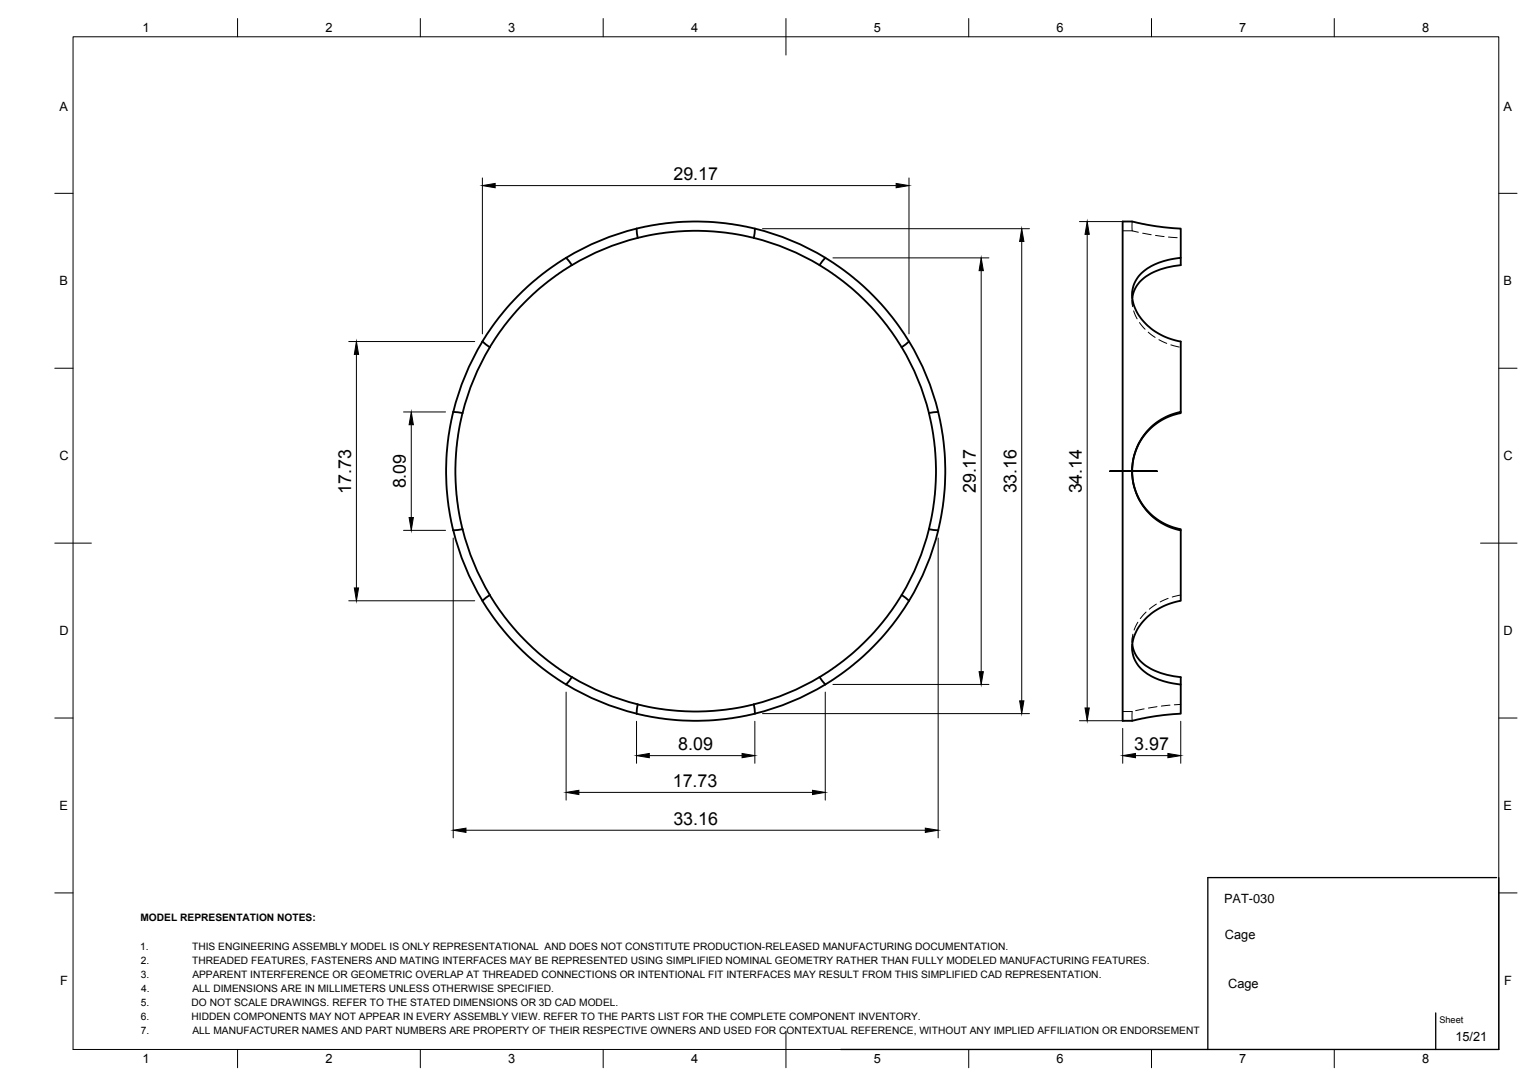
ISO-10303-21;
HEADER;
/* Generated by software containing ST-Developer
 * from STEP Tools, Inc. (www.steptools.com) 
 */

FILE_DESCRIPTION(
/* description */ ('Double-bearing flanged cartridge'),
/* implementation_level */ '2;1');

FILE_NAME(
/* name */ 'Cage.step',
/* time_stamp */ '2026-10-28T03:26:40-07:00',
/* author */ (''),
/* organization */ (''),
/* preprocessor_version */ 'ST-DEVELOPER v20.2',
/* originating_system */ 'Autodesk Translation Framework v15.17.0.0',
/* authorisation */ '');

FILE_SCHEMA (('AUTOMOTIVE_DESIGN { 1 0 10303 214 3 1 1 }'));
ENDSEC;

DATA;
#10=MECHANICAL_DESIGN_GEOMETRIC_PRESENTATION_REPRESENTATION('',(#201),#5535);
#116=B_SPLINE_CURVE_WITH_KNOTS('',3,(#3902,#3903,#3904,#3905,#3906,#3907,
#3908,#3909,#3910,#3911,#3912,#3913,#3914,#3915,#3916,#3917,#3918,#3919,
#3920,#3921,#3922,#3923),.UNSPECIFIED.,.F.,.F.,(4,2,2,2,2,2,2,2,2,2,4),
(0.0789094028588958,0.210573405340968,0.315860108011452,0.421146810681936,
0.522142632548711,0.623138454415485,0.72413427628226,0.825130098149035,
0.930416800819519,1.03570350349,1.16736750597208),.UNSPECIFIED.);
#117=B_SPLINE_CURVE_WITH_KNOTS('',3,(#3927,#3928,#3929,#3930,#3931,#3932,
#3933,#3934,#3935,#3936,#3937,#3938,#3939,#3940,#3941,#3942,#3943,#3944,
#3945,#3946,#3947,#3948),.UNSPECIFIED.,.F.,.F.,(4,2,2,2,2,2,2,2,2,2,4),
(0.0774793363974613,0.142088896491891,0.284177792983782,0.411119756996526,
0.514392970548519,0.617666184100513,0.720939397652506,0.8242126112045,0.951154575217244,
1.09324347170913,1.15785303180356),.UNSPECIFIED.);
#118=B_SPLINE_CURVE_WITH_KNOTS('',3,(#3954,#3955,#3956,#3957,#3958,#3959,
#3960,#3961,#3962,#3963,#3964,#3965,#3966,#3967,#3968,#3969,#3970,#3971,
#3972,#3973,#3974,#3975),.UNSPECIFIED.,.F.,.F.,(4,2,2,2,2,2,2,2,2,2,4),
(0.0774793363974613,0.142088896491891,0.284177792983782,0.411119756996525,
0.514392970548519,0.617666184100513,0.720939397652506,0.8242126112045,0.951154575217243,
1.09324347170913,1.15785303180356),.UNSPECIFIED.);
#119=B_SPLINE_CURVE_WITH_KNOTS('',3,(#3979,#3980,#3981,#3982,#3983,#3984,
#3985,#3986,#3987,#3988,#3989,#3990,#3991,#3992,#3993,#3994,#3995,#3996,
#3997,#3998,#3999,#4000),.UNSPECIFIED.,.F.,.F.,(4,2,2,2,2,2,2,2,2,2,4),
(0.0774793363974614,0.142088896491891,0.284177792983781,0.411119756996525,
0.514392970548519,0.617666184100512,0.720939397652506,0.824212611204499,
0.951154575217243,1.09324347170913,1.15785303180356),.UNSPECIFIED.);
#120=B_SPLINE_CURVE_WITH_KNOTS('',3,(#4004,#4005,#4006,#4007,#4008,#4009,
#4010,#4011,#4012,#4013,#4014,#4015),.UNSPECIFIED.,.F.,.F.,(4,2,2,2,2,4),
(0.0774793363974613,0.142088896491891,0.284177792983781,0.411119756996525,
0.514392970548519,0.617666184100512),.UNSPECIFIED.);
#121=B_SPLINE_CURVE_WITH_KNOTS('',3,(#4020,#4021,#4022,#4023,#4024,#4025,
#4026,#4027,#4028,#4029,#4030,#4031),.UNSPECIFIED.,.F.,.F.,(4,2,2,2,2,4),
(0.617666184100512,0.720939397652506,0.824212611204499,0.951154575217243,
1.09324347170913,1.15785303180356),.UNSPECIFIED.);
#122=B_SPLINE_CURVE_WITH_KNOTS('',3,(#4035,#4036,#4037,#4038,#4039,#4040,
#4041,#4042,#4043,#4044,#4045,#4046,#4047,#4048,#4049,#4050,#4051,#4052,
#4053,#4054,#4055,#4056),.UNSPECIFIED.,.F.,.F.,(4,2,2,2,2,2,2,2,2,2,4),
(0.0774793363974613,0.142088896491891,0.284177792983782,0.411119756996526,
0.514392970548519,0.617666184100513,0.720939397652507,0.8242126112045,0.951154575217245,
1.09324347170914,1.15785303180356),.UNSPECIFIED.);
#123=B_SPLINE_CURVE_WITH_KNOTS('',3,(#4060,#4061,#4062,#4063,#4064,#4065,
#4066,#4067,#4068,#4069,#4070,#4071,#4072,#4073,#4074,#4075,#4076,#4077,
#4078,#4079,#4080,#4081),.UNSPECIFIED.,.F.,.F.,(4,2,2,2,2,2,2,2,2,2,4),
(0.0774793363974613,0.142088896491891,0.284177792983782,0.411119756996526,
0.514392970548519,0.617666184100513,0.720939397652506,0.824212611204499,
0.951154575217243,1.09324347170913,1.15785303180356),.UNSPECIFIED.);
#124=B_SPLINE_CURVE_WITH_KNOTS('',3,(#4085,#4086,#4087,#4088,#4089,#4090,
#4091,#4092,#4093,#4094,#4095,#4096,#4097,#4098,#4099,#4100,#4101,#4102,
#4103,#4104,#4105,#4106),.UNSPECIFIED.,.F.,.F.,(4,2,2,2,2,2,2,2,2,2,4),
(0.0774793363974613,0.142088896491891,0.284177792983782,0.411119756996526,
0.514392970548519,0.617666184100513,0.720939397652506,0.8242126112045,0.951154575217244,
1.09324347170913,1.15785303180356),.UNSPECIFIED.);
#125=B_SPLINE_CURVE_WITH_KNOTS('',3,(#4110,#4111,#4112,#4113,#4114,#4115,
#4116,#4117,#4118,#4119,#4120,#4121,#4122,#4123,#4124,#4125,#4126,#4127,
#4128,#4129,#4130,#4131),.UNSPECIFIED.,.F.,.F.,(4,2,2,2,2,2,2,2,2,2,4),
(0.0774793363974613,0.142088896491891,0.284177792983782,0.411119756996526,
0.514392970548519,0.617666184100513,0.720939397652506,0.8242126112045,0.951154575217243,
1.09324347170913,1.15785303180356),.UNSPECIFIED.);
#126=B_SPLINE_CURVE_WITH_KNOTS('',3,(#4139,#4140,#4141,#4142,#4143,#4144,
#4145,#4146,#4147,#4148,#4149,#4150,#4151,#4152,#4153,#4154,#4155,#4156,
#4157,#4158,#4159,#4160),.UNSPECIFIED.,.F.,.F.,(4,2,2,2,2,2,2,2,2,2,4),
(0.0789094028588958,0.210573405340968,0.315860108011452,0.421146810681936,
0.522142632548711,0.623138454415485,0.72413427628226,0.825130098149035,
0.930416800819519,1.03570350349,1.16736750597208),.UNSPECIFIED.);
#127=B_SPLINE_CURVE_WITH_KNOTS('',3,(#4168,#4169,#4170,#4171,#4172,#4173,
#4174,#4175,#4176,#4177,#4178,#4179,#4180,#4181,#4182,#4183,#4184,#4185,
#4186,#4187,#4188,#4189),.UNSPECIFIED.,.F.,.F.,(4,2,2,2,2,2,2,2,2,2,4),
(0.0789094028588958,0.210573405340969,0.315860108011453,0.421146810681937,
0.522142632548712,0.623138454415486,0.724134276282261,0.825130098149035,
0.930416800819519,1.03570350349,1.16736750597208),.UNSPECIFIED.);
#128=B_SPLINE_CURVE_WITH_KNOTS('',3,(#4198,#4199,#4200,#4201,#4202,#4203,
#4204,#4205,#4206,#4207,#4208,#4209),.UNSPECIFIED.,.F.,.F.,(4,2,2,2,2,4),
(0.0789094028588958,0.210573405340968,0.315860108011452,0.421146810681937,
0.522142632548711,0.623138454415486),.UNSPECIFIED.);
#129=B_SPLINE_CURVE_WITH_KNOTS('',3,(#4211,#4212,#4213,#4214,#4215,#4216,
#4217,#4218,#4219,#4220,#4221,#4222),.UNSPECIFIED.,.F.,.F.,(4,2,2,2,2,4),
(0.623138454415486,0.72413427628226,0.825130098149035,0.930416800819519,
1.03570350349,1.16736750597208),.UNSPECIFIED.);
#130=B_SPLINE_CURVE_WITH_KNOTS('',3,(#4229,#4230,#4231,#4232,#4233,#4234,
#4235,#4236,#4237,#4238,#4239,#4240,#4241,#4242,#4243,#4244,#4245,#4246,
#4247,#4248,#4249,#4250),.UNSPECIFIED.,.F.,.F.,(4,2,2,2,2,2,2,2,2,2,4),
(0.0789094028588958,0.210573405340968,0.315860108011452,0.421146810681936,
0.522142632548711,0.623138454415486,0.72413427628226,0.825130098149035,
0.930416800819519,1.03570350349,1.16736750597208),.UNSPECIFIED.);
#131=B_SPLINE_CURVE_WITH_KNOTS('',3,(#4258,#4259,#4260,#4261,#4262,#4263,
#4264,#4265,#4266,#4267,#4268,#4269,#4270,#4271,#4272,#4273,#4274,#4275,
#4276,#4277,#4278,#4279),.UNSPECIFIED.,.F.,.F.,(4,2,2,2,2,2,2,2,2,2,4),
(0.0789094028588957,0.210573405340968,0.315860108011452,0.421146810681936,
0.522142632548711,0.623138454415485,0.72413427628226,0.825130098149035,
0.930416800819519,1.03570350349,1.16736750597207),.UNSPECIFIED.);
#132=B_SPLINE_CURVE_WITH_KNOTS('',3,(#4287,#4288,#4289,#4290,#4291,#4292,
#4293,#4294,#4295,#4296,#4297,#4298,#4299,#4300,#4301,#4302,#4303,#4304,
#4305,#4306,#4307,#4308),.UNSPECIFIED.,.F.,.F.,(4,2,2,2,2,2,2,2,2,2,4),
(0.0789094028588958,0.210573405340968,0.315860108011452,0.421146810681936,
0.522142632548711,0.623138454415486,0.72413427628226,0.825130098149035,
0.930416800819519,1.03570350349,1.16736750597208),.UNSPECIFIED.);
#133=B_SPLINE_CURVE_WITH_KNOTS('',3,(#4317,#4318,#4319,#4320,#4321,#4322,
#4323,#4324,#4325,#4326,#4327,#4328,#4329,#4330,#4331,#4332,#4333,#4334,
#4335,#4336,#4337,#4338),.UNSPECIFIED.,.F.,.F.,(4,2,2,2,2,2,2,2,2,2,4),
(0.0789094028588958,0.210573405340968,0.315860108011452,0.421146810681936,
0.522142632548711,0.623138454415485,0.72413427628226,0.825130098149035,
0.930416800819519,1.03570350349,1.16736750597208),.UNSPECIFIED.);
#144=SPHERICAL_SURFACE('',#2624,0.412776);
#145=SPHERICAL_SURFACE('',#2640,0.412776);
#146=SPHERICAL_SURFACE('',#2645,0.412776);
#147=SPHERICAL_SURFACE('',#2650,0.412776);
#148=SPHERICAL_SURFACE('',#2655,0.412776);
#149=SPHERICAL_SURFACE('',#2660,0.412776);
#150=SPHERICAL_SURFACE('',#2665,0.412776);
#151=SPHERICAL_SURFACE('',#2673,0.412776);
#166=SHAPE_REPRESENTATION_RELATIONSHIP('SRR','None',#5608,#180);
#180=ADVANCED_BREP_SHAPE_REPRESENTATION('',(#223),#5524);
#201=STYLED_ITEM('',(#5764),#223);
#223=MANIFOLD_SOLID_BREP('Continuous crown cage',#2335);
#257=FACE_BOUND('',#604,.T.);
#316=PLANE('',#2637);
#317=PLANE('',#2642);
#318=PLANE('',#2647);
#319=PLANE('',#2652);
#320=PLANE('',#2657);
#321=PLANE('',#2662);
#322=PLANE('',#2671);
#323=PLANE('',#2675);
#324=PLANE('',#2676);
#413=FACE_OUTER_BOUND('',#586,.T.);
#414=FACE_OUTER_BOUND('',#587,.T.);
#415=FACE_OUTER_BOUND('',#588,.T.);
#416=FACE_OUTER_BOUND('',#589,.T.);
#417=FACE_OUTER_BOUND('',#590,.T.);
#418=FACE_OUTER_BOUND('',#591,.T.);
#419=FACE_OUTER_BOUND('',#592,.T.);
#420=FACE_OUTER_BOUND('',#593,.T.);
#421=FACE_OUTER_BOUND('',#594,.T.);
#422=FACE_OUTER_BOUND('',#595,.T.);
#423=FACE_OUTER_BOUND('',#596,.T.);
#424=FACE_OUTER_BOUND('',#597,.T.);
#425=FACE_OUTER_BOUND('',#598,.T.);
#426=FACE_OUTER_BOUND('',#599,.T.);
#427=FACE_OUTER_BOUND('',#600,.T.);
#428=FACE_OUTER_BOUND('',#601,.T.);
#429=FACE_OUTER_BOUND('',#602,.T.);
#430=FACE_OUTER_BOUND('',#603,.T.);
#431=FACE_OUTER_BOUND('',#605,.T.);
#586=EDGE_LOOP('',(#1726,#1727,#1728,#1729));
#587=EDGE_LOOP('',(#1730,#1731,#1732,#1733,#1734,#1735,#1736,#1737,#1738,
#1739,#1740,#1741,#1742,#1743,#1744,#1745,#1746,#1747,#1748,#1749));
#588=EDGE_LOOP('',(#1750,#1751,#1752,#1753));
#589=EDGE_LOOP('',(#1754,#1755,#1756,#1757));
#590=EDGE_LOOP('',(#1758,#1759,#1760,#1761));
#591=EDGE_LOOP('',(#1762,#1763,#1764,#1765));
#592=EDGE_LOOP('',(#1766,#1767,#1768,#1769));
#593=EDGE_LOOP('',(#1770,#1771,#1772,#1773,#1774,#1775));
#594=EDGE_LOOP('',(#1776,#1777,#1778,#1779));
#595=EDGE_LOOP('',(#1780,#1781,#1782,#1783));
#596=EDGE_LOOP('',(#1784,#1785,#1786,#1787));
#597=EDGE_LOOP('',(#1788,#1789,#1790,#1791));
#598=EDGE_LOOP('',(#1792,#1793,#1794,#1795));
#599=EDGE_LOOP('',(#1796,#1797,#1798,#1799));
#600=EDGE_LOOP('',(#1800,#1801,#1802,#1803,#1804,#1805,#1806,#1807,#1808,
#1809,#1810,#1811,#1812,#1813,#1814,#1815,#1816,#1817,#1818,#1819));
#601=EDGE_LOOP('',(#1820,#1821,#1822,#1823));
#602=EDGE_LOOP('',(#1824,#1825,#1826,#1827));
#603=EDGE_LOOP('',(#1828));
#604=EDGE_LOOP('',(#1829));
#605=EDGE_LOOP('',(#1830,#1831,#1832,#1833));
#752=LINE('',#4017,#838);
#753=LINE('',#4313,#839);
#838=VECTOR('',#3151,1.706752);
#839=VECTOR('',#3228,1.643248);
#960=CIRCLE('',#2625,0.405071403305639);
#961=CIRCLE('',#2626,0.405071403305639);
#962=CIRCLE('',#2628,1.706752);
#963=CIRCLE('',#2629,1.706752);
#964=CIRCLE('',#2630,1.706752);
#965=CIRCLE('',#2631,1.706752);
#966=CIRCLE('',#2632,1.706752);
#967=CIRCLE('',#2633,1.706752);
#968=CIRCLE('',#2634,1.706752);
#969=CIRCLE('',#2635,1.706752);
#970=CIRCLE('',#2636,1.706752);
#971=CIRCLE('',#2638,1.643248);
#972=CIRCLE('',#2639,0.405071403305639);
#973=CIRCLE('',#2641,0.405071403305639);
#974=CIRCLE('',#2643,1.643248);
#975=CIRCLE('',#2644,0.405071403305639);
#976=CIRCLE('',#2646,0.405071403305639);
#977=CIRCLE('',#2648,1.643248);
#978=CIRCLE('',#2649,0.405071403305639);
#979=CIRCLE('',#2651,0.405071403305639);
#980=CIRCLE('',#2653,1.643248);
#981=CIRCLE('',#2654,0.405071403305639);
#982=CIRCLE('',#2656,0.405071403305639);
#983=CIRCLE('',#2658,1.643248);
#984=CIRCLE('',#2659,0.405071403305639);
#985=CIRCLE('',#2661,0.405071403305639);
#986=CIRCLE('',#2663,1.643248);
#987=CIRCLE('',#2664,0.405071403305639);
#988=CIRCLE('',#2666,0.405071403305639);
#989=CIRCLE('',#2668,1.643248);
#990=CIRCLE('',#2669,1.643248);
#991=CIRCLE('',#2670,1.643248);
#992=CIRCLE('',#2672,0.405071403305639);
#993=CIRCLE('',#2674,0.405071403305639);
#1140=VERTEX_POINT('',#3900);
#1141=VERTEX_POINT('',#3901);
#1142=VERTEX_POINT('',#3924);
#1143=VERTEX_POINT('',#3926);
#1144=VERTEX_POINT('',#3951);
#1145=VERTEX_POINT('',#3953);
#1146=VERTEX_POINT('',#3976);
#1147=VERTEX_POINT('',#3978);
#1148=VERTEX_POINT('',#4001);
#1149=VERTEX_POINT('',#4003);
#1150=VERTEX_POINT('',#4016);
#1151=VERTEX_POINT('',#4019);
#1152=VERTEX_POINT('',#4032);
#1153=VERTEX_POINT('',#4034);
#1154=VERTEX_POINT('',#4057);
#1155=VERTEX_POINT('',#4059);
#1156=VERTEX_POINT('',#4082);
#1157=VERTEX_POINT('',#4084);
#1158=VERTEX_POINT('',#4107);
#1159=VERTEX_POINT('',#4109);
#1160=VERTEX_POINT('',#4134);
#1161=VERTEX_POINT('',#4138);
#1162=VERTEX_POINT('',#4163);
#1163=VERTEX_POINT('',#4167);
#1164=VERTEX_POINT('',#4192);
#1165=VERTEX_POINT('',#4196);
#1166=VERTEX_POINT('',#4197);
#1167=VERTEX_POINT('',#4224);
#1168=VERTEX_POINT('',#4228);
#1169=VERTEX_POINT('',#4253);
#1170=VERTEX_POINT('',#4257);
#1171=VERTEX_POINT('',#4282);
#1172=VERTEX_POINT('',#4286);
#1173=VERTEX_POINT('',#4311);
#1174=VERTEX_POINT('',#4314);
#1175=VERTEX_POINT('',#4316);
#1356=EDGE_CURVE('',#1140,#1141,#116,.T.);
#1357=EDGE_CURVE('',#1142,#1140,#960,.T.);
#1358=EDGE_CURVE('',#1143,#1142,#117,.T.);
#1359=EDGE_CURVE('',#1141,#1143,#961,.T.);
#1360=EDGE_CURVE('',#1144,#1142,#962,.T.);
#1361=EDGE_CURVE('',#1144,#1145,#118,.T.);
#1362=EDGE_CURVE('',#1146,#1145,#963,.T.);
#1363=EDGE_CURVE('',#1146,#1147,#119,.T.);
#1364=EDGE_CURVE('',#1148,#1147,#964,.T.);
#1365=EDGE_CURVE('',#1148,#1149,#120,.T.);
#1366=EDGE_CURVE('',#1149,#1150,#752,.T.);
#1367=EDGE_CURVE('',#1150,#1150,#965,.T.);
#1368=EDGE_CURVE('',#1149,#1151,#121,.T.);
#1369=EDGE_CURVE('',#1152,#1151,#966,.T.);
#1370=EDGE_CURVE('',#1152,#1153,#122,.T.);
#1371=EDGE_CURVE('',#1154,#1153,#967,.T.);
#1372=EDGE_CURVE('',#1154,#1155,#123,.T.);
#1373=EDGE_CURVE('',#1156,#1155,#968,.T.);
#1374=EDGE_CURVE('',#1156,#1157,#124,.T.);
#1375=EDGE_CURVE('',#1158,#1157,#969,.T.);
#1376=EDGE_CURVE('',#1158,#1159,#125,.T.);
#1377=EDGE_CURVE('',#1143,#1159,#970,.T.);
#1378=EDGE_CURVE('',#1140,#1160,#971,.T.);
#1379=EDGE_CURVE('',#1160,#1144,#972,.T.);
#1380=EDGE_CURVE('',#1161,#1160,#126,.T.);
#1381=EDGE_CURVE('',#1145,#1161,#973,.T.);
#1382=EDGE_CURVE('',#1161,#1162,#974,.T.);
#1383=EDGE_CURVE('',#1162,#1146,#975,.T.);
#1384=EDGE_CURVE('',#1163,#1162,#127,.T.);
#1385=EDGE_CURVE('',#1147,#1163,#976,.T.);
#1386=EDGE_CURVE('',#1163,#1164,#977,.T.);
#1387=EDGE_CURVE('',#1164,#1148,#978,.T.);
#1388=EDGE_CURVE('',#1165,#1166,#128,.T.);
#1389=EDGE_CURVE('',#1151,#1165,#979,.T.);
#1390=EDGE_CURVE('',#1166,#1164,#129,.T.);
#1391=EDGE_CURVE('',#1165,#1167,#980,.T.);
#1392=EDGE_CURVE('',#1167,#1152,#981,.T.);
#1393=EDGE_CURVE('',#1168,#1167,#130,.T.);
#1394=EDGE_CURVE('',#1153,#1168,#982,.T.);
#1395=EDGE_CURVE('',#1168,#1169,#983,.T.);
#1396=EDGE_CURVE('',#1169,#1154,#984,.T.);
#1397=EDGE_CURVE('',#1170,#1169,#131,.T.);
#1398=EDGE_CURVE('',#1155,#1170,#985,.T.);
#1399=EDGE_CURVE('',#1170,#1171,#986,.T.);
#1400=EDGE_CURVE('',#1171,#1156,#987,.T.);
#1401=EDGE_CURVE('',#1172,#1171,#132,.T.);
#1402=EDGE_CURVE('',#1157,#1172,#988,.T.);
#1403=EDGE_CURVE('',#1173,#1173,#989,.T.);
#1404=EDGE_CURVE('',#1173,#1166,#753,.T.);
#1405=EDGE_CURVE('',#1174,#1141,#990,.T.);
#1406=EDGE_CURVE('',#1174,#1175,#133,.T.);
#1407=EDGE_CURVE('',#1172,#1175,#991,.T.);
#1408=EDGE_CURVE('',#1159,#1174,#992,.T.);
#1409=EDGE_CURVE('',#1175,#1158,#993,.T.);
#1726=ORIENTED_EDGE('',*,*,#1356,.F.);
#1727=ORIENTED_EDGE('',*,*,#1357,.F.);
#1728=ORIENTED_EDGE('',*,*,#1358,.F.);
#1729=ORIENTED_EDGE('',*,*,#1359,.F.);
#1730=ORIENTED_EDGE('',*,*,#1358,.T.);
#1731=ORIENTED_EDGE('',*,*,#1360,.F.);
#1732=ORIENTED_EDGE('',*,*,#1361,.T.);
#1733=ORIENTED_EDGE('',*,*,#1362,.F.);
#1734=ORIENTED_EDGE('',*,*,#1363,.T.);
#1735=ORIENTED_EDGE('',*,*,#1364,.F.);
#1736=ORIENTED_EDGE('',*,*,#1365,.T.);
#1737=ORIENTED_EDGE('',*,*,#1366,.T.);
#1738=ORIENTED_EDGE('',*,*,#1367,.F.);
#1739=ORIENTED_EDGE('',*,*,#1366,.F.);
#1740=ORIENTED_EDGE('',*,*,#1368,.T.);
#1741=ORIENTED_EDGE('',*,*,#1369,.F.);
#1742=ORIENTED_EDGE('',*,*,#1370,.T.);
#1743=ORIENTED_EDGE('',*,*,#1371,.F.);
#1744=ORIENTED_EDGE('',*,*,#1372,.T.);
#1745=ORIENTED_EDGE('',*,*,#1373,.F.);
#1746=ORIENTED_EDGE('',*,*,#1374,.T.);
#1747=ORIENTED_EDGE('',*,*,#1375,.F.);
#1748=ORIENTED_EDGE('',*,*,#1376,.T.);
#1749=ORIENTED_EDGE('',*,*,#1377,.F.);
#1750=ORIENTED_EDGE('',*,*,#1357,.T.);
#1751=ORIENTED_EDGE('',*,*,#1378,.T.);
#1752=ORIENTED_EDGE('',*,*,#1379,.T.);
#1753=ORIENTED_EDGE('',*,*,#1360,.T.);
#1754=ORIENTED_EDGE('',*,*,#1380,.F.);
#1755=ORIENTED_EDGE('',*,*,#1381,.F.);
#1756=ORIENTED_EDGE('',*,*,#1361,.F.);
#1757=ORIENTED_EDGE('',*,*,#1379,.F.);
#1758=ORIENTED_EDGE('',*,*,#1381,.T.);
#1759=ORIENTED_EDGE('',*,*,#1382,.T.);
#1760=ORIENTED_EDGE('',*,*,#1383,.T.);
#1761=ORIENTED_EDGE('',*,*,#1362,.T.);
#1762=ORIENTED_EDGE('',*,*,#1384,.F.);
#1763=ORIENTED_EDGE('',*,*,#1385,.F.);
#1764=ORIENTED_EDGE('',*,*,#1363,.F.);
#1765=ORIENTED_EDGE('',*,*,#1383,.F.);
#1766=ORIENTED_EDGE('',*,*,#1385,.T.);
#1767=ORIENTED_EDGE('',*,*,#1386,.T.);
#1768=ORIENTED_EDGE('',*,*,#1387,.T.);
#1769=ORIENTED_EDGE('',*,*,#1364,.T.);
#1770=ORIENTED_EDGE('',*,*,#1388,.F.);
#1771=ORIENTED_EDGE('',*,*,#1389,.F.);
#1772=ORIENTED_EDGE('',*,*,#1368,.F.);
#1773=ORIENTED_EDGE('',*,*,#1365,.F.);
#1774=ORIENTED_EDGE('',*,*,#1387,.F.);
#1775=ORIENTED_EDGE('',*,*,#1390,.F.);
#1776=ORIENTED_EDGE('',*,*,#1389,.T.);
#1777=ORIENTED_EDGE('',*,*,#1391,.T.);
#1778=ORIENTED_EDGE('',*,*,#1392,.T.);
#1779=ORIENTED_EDGE('',*,*,#1369,.T.);
#1780=ORIENTED_EDGE('',*,*,#1393,.F.);
#1781=ORIENTED_EDGE('',*,*,#1394,.F.);
#1782=ORIENTED_EDGE('',*,*,#1370,.F.);
#1783=ORIENTED_EDGE('',*,*,#1392,.F.);
#1784=ORIENTED_EDGE('',*,*,#1394,.T.);
#1785=ORIENTED_EDGE('',*,*,#1395,.T.);
#1786=ORIENTED_EDGE('',*,*,#1396,.T.);
#1787=ORIENTED_EDGE('',*,*,#1371,.T.);
#1788=ORIENTED_EDGE('',*,*,#1397,.F.);
#1789=ORIENTED_EDGE('',*,*,#1398,.F.);
#1790=ORIENTED_EDGE('',*,*,#1372,.F.);
#1791=ORIENTED_EDGE('',*,*,#1396,.F.);
#1792=ORIENTED_EDGE('',*,*,#1398,.T.);
#1793=ORIENTED_EDGE('',*,*,#1399,.T.);
#1794=ORIENTED_EDGE('',*,*,#1400,.T.);
#1795=ORIENTED_EDGE('',*,*,#1373,.T.);
#1796=ORIENTED_EDGE('',*,*,#1374,.F.);
#1797=ORIENTED_EDGE('',*,*,#1400,.F.);
#1798=ORIENTED_EDGE('',*,*,#1401,.F.);
#1799=ORIENTED_EDGE('',*,*,#1402,.F.);
#1800=ORIENTED_EDGE('',*,*,#1403,.F.);
#1801=ORIENTED_EDGE('',*,*,#1404,.T.);
#1802=ORIENTED_EDGE('',*,*,#1390,.T.);
#1803=ORIENTED_EDGE('',*,*,#1386,.F.);
#1804=ORIENTED_EDGE('',*,*,#1384,.T.);
#1805=ORIENTED_EDGE('',*,*,#1382,.F.);
#1806=ORIENTED_EDGE('',*,*,#1380,.T.);
#1807=ORIENTED_EDGE('',*,*,#1378,.F.);
#1808=ORIENTED_EDGE('',*,*,#1356,.T.);
#1809=ORIENTED_EDGE('',*,*,#1405,.F.);
#1810=ORIENTED_EDGE('',*,*,#1406,.T.);
#1811=ORIENTED_EDGE('',*,*,#1407,.F.);
#1812=ORIENTED_EDGE('',*,*,#1401,.T.);
#1813=ORIENTED_EDGE('',*,*,#1399,.F.);
#1814=ORIENTED_EDGE('',*,*,#1397,.T.);
#1815=ORIENTED_EDGE('',*,*,#1395,.F.);
#1816=ORIENTED_EDGE('',*,*,#1393,.T.);
#1817=ORIENTED_EDGE('',*,*,#1391,.F.);
#1818=ORIENTED_EDGE('',*,*,#1388,.T.);
#1819=ORIENTED_EDGE('',*,*,#1404,.F.);
#1820=ORIENTED_EDGE('',*,*,#1359,.T.);
#1821=ORIENTED_EDGE('',*,*,#1377,.T.);
#1822=ORIENTED_EDGE('',*,*,#1408,.T.);
#1823=ORIENTED_EDGE('',*,*,#1405,.T.);
#1824=ORIENTED_EDGE('',*,*,#1376,.F.);
#1825=ORIENTED_EDGE('',*,*,#1409,.F.);
#1826=ORIENTED_EDGE('',*,*,#1406,.F.);
#1827=ORIENTED_EDGE('',*,*,#1408,.F.);
#1828=ORIENTED_EDGE('',*,*,#1367,.T.);
#1829=ORIENTED_EDGE('',*,*,#1403,.T.);
#1830=ORIENTED_EDGE('',*,*,#1402,.T.);
#1831=ORIENTED_EDGE('',*,*,#1407,.T.);
#1832=ORIENTED_EDGE('',*,*,#1409,.T.);
#1833=ORIENTED_EDGE('',*,*,#1375,.T.);
#2136=CYLINDRICAL_SURFACE('',#2627,1.706752);
#2137=CYLINDRICAL_SURFACE('',#2667,1.643248);
#2227=ADVANCED_FACE('',(#413),#144,.F.);
#2228=ADVANCED_FACE('',(#414),#2136,.T.);
#2229=ADVANCED_FACE('',(#415),#316,.T.);
#2230=ADVANCED_FACE('',(#416),#145,.F.);
#2231=ADVANCED_FACE('',(#417),#317,.T.);
#2232=ADVANCED_FACE('',(#418),#146,.F.);
#2233=ADVANCED_FACE('',(#419),#318,.T.);
#2234=ADVANCED_FACE('',(#420),#147,.F.);
#2235=ADVANCED_FACE('',(#421),#319,.T.);
#2236=ADVANCED_FACE('',(#422),#148,.F.);
#2237=ADVANCED_FACE('',(#423),#320,.T.);
#2238=ADVANCED_FACE('',(#424),#149,.F.);
#2239=ADVANCED_FACE('',(#425),#321,.T.);
#2240=ADVANCED_FACE('',(#426),#150,.F.);
#2241=ADVANCED_FACE('',(#427),#2137,.F.);
#2242=ADVANCED_FACE('',(#428),#322,.T.);
#2243=ADVANCED_FACE('',(#429),#151,.F.);
#2244=ADVANCED_FACE('',(#430,#257),#323,.T.);
#2245=ADVANCED_FACE('',(#431),#324,.T.);
#2335=CLOSED_SHELL('',(#2227,#2228,#2229,#2230,#2231,#2232,#2233,#2234,
#2235,#2236,#2237,#2238,#2239,#2240,#2241,#2242,#2243,#2244,#2245));
#2623=AXIS2_PLACEMENT_3D('',#3898,#3135,#3136);
#2624=AXIS2_PLACEMENT_3D('',#3899,#3137,#3138);
#2625=AXIS2_PLACEMENT_3D('',#3925,#3139,#3140);
#2626=AXIS2_PLACEMENT_3D('',#3949,#3141,#3142);
#2627=AXIS2_PLACEMENT_3D('',#3950,#3143,#3144);
#2628=AXIS2_PLACEMENT_3D('',#3952,#3145,#3146);
#2629=AXIS2_PLACEMENT_3D('',#3977,#3147,#3148);
#2630=AXIS2_PLACEMENT_3D('',#4002,#3149,#3150);
#2631=AXIS2_PLACEMENT_3D('',#4018,#3152,#3153);
#2632=AXIS2_PLACEMENT_3D('',#4033,#3154,#3155);
#2633=AXIS2_PLACEMENT_3D('',#4058,#3156,#3157);
#2634=AXIS2_PLACEMENT_3D('',#4083,#3158,#3159);
#2635=AXIS2_PLACEMENT_3D('',#4108,#3160,#3161);
#2636=AXIS2_PLACEMENT_3D('',#4132,#3162,#3163);
#2637=AXIS2_PLACEMENT_3D('',#4133,#3164,#3165);
#2638=AXIS2_PLACEMENT_3D('',#4135,#3166,#3167);
#2639=AXIS2_PLACEMENT_3D('',#4136,#3168,#3169);
#2640=AXIS2_PLACEMENT_3D('',#4137,#3170,#3171);
#2641=AXIS2_PLACEMENT_3D('',#4161,#3172,#3173);
#2642=AXIS2_PLACEMENT_3D('',#4162,#3174,#3175);
#2643=AXIS2_PLACEMENT_3D('',#4164,#3176,#3177);
#2644=AXIS2_PLACEMENT_3D('',#4165,#3178,#3179);
#2645=AXIS2_PLACEMENT_3D('',#4166,#3180,#3181);
#2646=AXIS2_PLACEMENT_3D('',#4190,#3182,#3183);
#2647=AXIS2_PLACEMENT_3D('',#4191,#3184,#3185);
#2648=AXIS2_PLACEMENT_3D('',#4193,#3186,#3187);
#2649=AXIS2_PLACEMENT_3D('',#4194,#3188,#3189);
#2650=AXIS2_PLACEMENT_3D('',#4195,#3190,#3191);
#2651=AXIS2_PLACEMENT_3D('',#4210,#3192,#3193);
#2652=AXIS2_PLACEMENT_3D('',#4223,#3194,#3195);
#2653=AXIS2_PLACEMENT_3D('',#4225,#3196,#3197);
#2654=AXIS2_PLACEMENT_3D('',#4226,#3198,#3199);
#2655=AXIS2_PLACEMENT_3D('',#4227,#3200,#3201);
#2656=AXIS2_PLACEMENT_3D('',#4251,#3202,#3203);
#2657=AXIS2_PLACEMENT_3D('',#4252,#3204,#3205);
#2658=AXIS2_PLACEMENT_3D('',#4254,#3206,#3207);
#2659=AXIS2_PLACEMENT_3D('',#4255,#3208,#3209);
#2660=AXIS2_PLACEMENT_3D('',#4256,#3210,#3211);
#2661=AXIS2_PLACEMENT_3D('',#4280,#3212,#3213);
#2662=AXIS2_PLACEMENT_3D('',#4281,#3214,#3215);
#2663=AXIS2_PLACEMENT_3D('',#4283,#3216,#3217);
#2664=AXIS2_PLACEMENT_3D('',#4284,#3218,#3219);
#2665=AXIS2_PLACEMENT_3D('',#4285,#3220,#3221);
#2666=AXIS2_PLACEMENT_3D('',#4309,#3222,#3223);
#2667=AXIS2_PLACEMENT_3D('',#4310,#3224,#3225);
#2668=AXIS2_PLACEMENT_3D('',#4312,#3226,#3227);
#2669=AXIS2_PLACEMENT_3D('',#4315,#3229,#3230);
#2670=AXIS2_PLACEMENT_3D('',#4339,#3231,#3232);
#2671=AXIS2_PLACEMENT_3D('',#4340,#3233,#3234);
#2672=AXIS2_PLACEMENT_3D('',#4341,#3235,#3236);
#2673=AXIS2_PLACEMENT_3D('',#4342,#3237,#3238);
#2674=AXIS2_PLACEMENT_3D('',#4343,#3239,#3240);
#2675=AXIS2_PLACEMENT_3D('',#4344,#3241,#3242);
#2676=AXIS2_PLACEMENT_3D('',#4345,#3243,#3244);
#3135=DIRECTION('axis',(0.,0.,1.));
#3136=DIRECTION('refdir',(1.,0.,0.));
#3137=DIRECTION('center_axis',(0.,0.,1.));
#3138=DIRECTION('ref_axis',(1.,0.,0.));
#3139=DIRECTION('center_axis',(0.,-1.,0.));
#3140=DIRECTION('ref_axis',(0.,0.,-1.));
#3141=DIRECTION('center_axis',(0.,-1.,0.));
#3142=DIRECTION('ref_axis',(0.,0.,-1.));
#3143=DIRECTION('center_axis',(0.,1.,0.));
#3144=DIRECTION('ref_axis',(1.,0.,0.));
#3145=DIRECTION('center_axis',(0.,1.,0.));
#3146=DIRECTION('ref_axis',(1.,0.,0.));
#3147=DIRECTION('center_axis',(0.,1.,0.));
#3148=DIRECTION('ref_axis',(1.,0.,0.));
#3149=DIRECTION('center_axis',(0.,1.,0.));
#3150=DIRECTION('ref_axis',(1.,0.,0.));
#3151=DIRECTION('',(0.,-1.,0.));
#3152=DIRECTION('center_axis',(0.,-1.,0.));
#3153=DIRECTION('ref_axis',(1.,0.,0.));
#3154=DIRECTION('center_axis',(0.,1.,0.));
#3155=DIRECTION('ref_axis',(1.,0.,0.));
#3156=DIRECTION('center_axis',(0.,1.,0.));
#3157=DIRECTION('ref_axis',(1.,0.,0.));
#3158=DIRECTION('center_axis',(0.,1.,0.));
#3159=DIRECTION('ref_axis',(1.,0.,0.));
#3160=DIRECTION('center_axis',(0.,1.,0.));
#3161=DIRECTION('ref_axis',(1.,0.,0.));
#3162=DIRECTION('center_axis',(0.,1.,0.));
#3163=DIRECTION('ref_axis',(1.,0.,0.));
#3164=DIRECTION('center_axis',(0.,1.,0.));
#3165=DIRECTION('ref_axis',(1.,0.,0.));
#3166=DIRECTION('center_axis',(0.,-1.,0.));
#3167=DIRECTION('ref_axis',(1.,0.,0.));
#3168=DIRECTION('center_axis',(0.,-1.,0.));
#3169=DIRECTION('ref_axis',(0.,0.,-1.));
#3170=DIRECTION('center_axis',(6.12323399573677E-17,0.,1.));
#3171=DIRECTION('ref_axis',(1.,0.,0.));
#3172=DIRECTION('center_axis',(0.,-1.,0.));
#3173=DIRECTION('ref_axis',(0.,0.,-1.));
#3174=DIRECTION('center_axis',(0.,1.,0.));
#3175=DIRECTION('ref_axis',(1.,0.,0.));
#3176=DIRECTION('center_axis',(0.,-1.,0.));
#3177=DIRECTION('ref_axis',(1.,0.,0.));
#3178=DIRECTION('center_axis',(0.,-1.,0.));
#3179=DIRECTION('ref_axis',(0.,0.,-1.));
#3180=DIRECTION('center_axis',(0.,0.,1.));
#3181=DIRECTION('ref_axis',(1.,0.,0.));
#3182=DIRECTION('center_axis',(0.,-1.,0.));
#3183=DIRECTION('ref_axis',(0.,0.,-1.));
#3184=DIRECTION('center_axis',(0.,1.,0.));
#3185=DIRECTION('ref_axis',(1.,0.,0.));
#3186=DIRECTION('center_axis',(0.,-1.,0.));
#3187=DIRECTION('ref_axis',(1.,0.,0.));
#3188=DIRECTION('center_axis',(0.,-1.,0.));
#3189=DIRECTION('ref_axis',(0.,0.,-1.));
#3190=DIRECTION('center_axis',(0.,0.,1.));
#3191=DIRECTION('ref_axis',(1.,0.,0.));
#3192=DIRECTION('center_axis',(0.,-1.,0.));
#3193=DIRECTION('ref_axis',(0.,0.,-1.));
#3194=DIRECTION('center_axis',(0.,1.,0.));
#3195=DIRECTION('ref_axis',(1.,0.,0.));
#3196=DIRECTION('center_axis',(0.,-1.,0.));
#3197=DIRECTION('ref_axis',(1.,0.,0.));
#3198=DIRECTION('center_axis',(0.,-1.,0.));
#3199=DIRECTION('ref_axis',(0.,0.,-1.));
#3200=DIRECTION('center_axis',(0.,0.,1.));
#3201=DIRECTION('ref_axis',(1.,0.,0.));
#3202=DIRECTION('center_axis',(0.,-1.,0.));
#3203=DIRECTION('ref_axis',(0.,0.,-1.));
#3204=DIRECTION('center_axis',(0.,1.,0.));
#3205=DIRECTION('ref_axis',(1.,0.,0.));
#3206=DIRECTION('center_axis',(0.,-1.,0.));
#3207=DIRECTION('ref_axis',(1.,0.,0.));
#3208=DIRECTION('center_axis',(0.,-1.,0.));
#3209=DIRECTION('ref_axis',(0.,0.,-1.));
#3210=DIRECTION('center_axis',(6.12323399573676E-17,0.,1.));
#3211=DIRECTION('ref_axis',(1.,0.,0.));
#3212=DIRECTION('center_axis',(0.,-1.,0.));
#3213=DIRECTION('ref_axis',(0.,0.,-1.));
#3214=DIRECTION('center_axis',(0.,1.,0.));
#3215=DIRECTION('ref_axis',(1.,0.,0.));
#3216=DIRECTION('center_axis',(0.,-1.,0.));
#3217=DIRECTION('ref_axis',(1.,0.,0.));
#3218=DIRECTION('center_axis',(0.,-1.,0.));
#3219=DIRECTION('ref_axis',(0.,0.,-1.));
#3220=DIRECTION('center_axis',(0.,0.,1.));
#3221=DIRECTION('ref_axis',(1.,0.,0.));
#3222=DIRECTION('center_axis',(0.,-1.,0.));
#3223=DIRECTION('ref_axis',(0.,0.,-1.));
#3224=DIRECTION('center_axis',(0.,1.,0.));
#3225=DIRECTION('ref_axis',(1.,0.,0.));
#3226=DIRECTION('center_axis',(0.,1.,0.));
#3227=DIRECTION('ref_axis',(1.,0.,0.));
#3228=DIRECTION('',(0.,1.,0.));
#3229=DIRECTION('center_axis',(0.,-1.,0.));
#3230=DIRECTION('ref_axis',(1.,0.,0.));
#3231=DIRECTION('center_axis',(0.,-1.,0.));
#3232=DIRECTION('ref_axis',(1.,0.,0.));
#3233=DIRECTION('center_axis',(0.,1.,0.));
#3234=DIRECTION('ref_axis',(1.,0.,0.));
#3235=DIRECTION('center_axis',(0.,-1.,0.));
#3236=DIRECTION('ref_axis',(0.,0.,-1.));
#3237=DIRECTION('center_axis',(0.,0.,1.));
#3238=DIRECTION('ref_axis',(1.,0.,0.));
#3239=DIRECTION('center_axis',(0.,-1.,0.));
#3240=DIRECTION('ref_axis',(0.,0.,-1.));
#3241=DIRECTION('center_axis',(0.,-1.,0.));
#3242=DIRECTION('ref_axis',(-1.,0.,0.));
#3243=DIRECTION('center_axis',(0.,1.,0.));
#3244=DIRECTION('ref_axis',(1.,0.,0.));
#3898=CARTESIAN_POINT('',(0.,0.,0.));
#3899=CARTESIAN_POINT('Origin',(1.18440385848747,0.,1.18440385848747));
#3900=CARTESIAN_POINT('',(0.846804978391753,-0.07938,1.40825612658882));
#3901=CARTESIAN_POINT('',(1.40825612658882,-0.07938,0.846804978391754));
#3902=CARTESIAN_POINT('Ctrl Pts',(0.846804978391752,-0.0793800000000001,
1.40825612658882));
#3903=CARTESIAN_POINT('Ctrl Pts',(0.854205272175554,-0.123401821157026,
1.40380622184538));
#3904=CARTESIAN_POINT('Ctrl Pts',(0.867957148219441,-0.166543350814306,
1.39550172959303));
#3905=CARTESIAN_POINT('Ctrl Pts',(0.902193646979982,-0.237231147975234,
1.3735491215176));
#3906=CARTESIAN_POINT('Ctrl Pts',(0.920778333482564,-0.266264900654909,
1.36127834356734));
#3907=CARTESIAN_POINT('Ctrl Pts',(0.962485392528369,-0.317195968905306,
1.33211611256184));
#3908=CARTESIAN_POINT('Ctrl Pts',(0.985600426557816,-0.33909093068465,1.31521005565926));
#3909=CARTESIAN_POINT('Ctrl Pts',(1.03253285680459,-0.373586846396559,1.27866649102984));
#3910=CARTESIAN_POINT('Ctrl Pts',(1.05871835910697,-0.388086240756494,1.25722555095714));
#3911=CARTESIAN_POINT('Ctrl Pts',(1.11153475808518,-0.407068917407805,1.2107812086231));
#3912=CARTESIAN_POINT('Ctrl Pts',(1.13814686046673,-0.411552957311693,1.18575674747573));
#3913=CARTESIAN_POINT('Ctrl Pts',(1.18575674747573,-0.411552957311693,1.13814686046673));
#3914=CARTESIAN_POINT('Ctrl Pts',(1.2107812086231,-0.407068917407805,1.11153475808518));
#3915=CARTESIAN_POINT('Ctrl Pts',(1.25722555095713,-0.388086240756494,1.05871835910697));
#3916=CARTESIAN_POINT('Ctrl Pts',(1.27866649102984,-0.373586846396559,1.03253285680459));
#3917=CARTESIAN_POINT('Ctrl Pts',(1.31521005565926,-0.33909093068465,0.985600426557816));
#3918=CARTESIAN_POINT('Ctrl Pts',(1.33211611256184,-0.317195968905306,0.962485392528369));
#3919=CARTESIAN_POINT('Ctrl Pts',(1.36127834356734,-0.266264900654909,0.920778333482565));
#3920=CARTESIAN_POINT('Ctrl Pts',(1.3735491215176,-0.237231147975234,0.902193646979983));
#3921=CARTESIAN_POINT('Ctrl Pts',(1.39550172959303,-0.166543350814306,0.867957148219442));
#3922=CARTESIAN_POINT('Ctrl Pts',(1.40380622184538,-0.123401821157026,0.854205272175555));
#3923=CARTESIAN_POINT('Ctrl Pts',(1.40825612658882,-0.0793800000000001,
0.846804978391753));
#3924=CARTESIAN_POINT('',(0.886256117232623,-0.07938,1.45861320581289));
#3925=CARTESIAN_POINT('Origin',(1.18440385848747,-0.07938,1.18440385848747));
#3926=CARTESIAN_POINT('',(1.45861320581289,-0.07938,0.886256117232624));
#3927=CARTESIAN_POINT('Ctrl Pts',(1.45861320581289,-0.0793800000000001,
0.886256117232623));
#3928=CARTESIAN_POINT('Ctrl Pts',(1.45630208793976,-0.101649918886749,0.890059788636852));
#3929=CARTESIAN_POINT('Ctrl Pts',(1.45296717977858,-0.123823518623746,0.895520212222107));
#3930=CARTESIAN_POINT('Ctrl Pts',(1.43904931717599,-0.192480977588836,0.917859913453975));
#3931=CARTESIAN_POINT('Ctrl Pts',(1.4243271592157,-0.236152929235938,0.940896403863072));
#3932=CARTESIAN_POINT('Ctrl Pts',(1.39055359345152,-0.303141259068212,0.990027513266106));
#3933=CARTESIAN_POINT('Ctrl Pts',(1.36743459453896,-0.335108247315849,1.02199477007745));
#3934=CARTESIAN_POINT('Ctrl Pts',(1.32643091652006,-0.373243761060364,1.07446535104584));
#3935=CARTESIAN_POINT('Ctrl Pts',(1.30441816675528,-0.387888272594439,1.10126842659597));
#3936=CARTESIAN_POINT('Ctrl Pts',(1.25681160160691,-0.407041111792943,1.15530234155453));
#3937=CARTESIAN_POINT('Ctrl Pts',(1.23119764287622,-0.411552957311693,1.18251418313119));
#3938=CARTESIAN_POINT('Ctrl Pts',(1.18251418313119,-0.411552957311693,1.23119764287622));
#3939=CARTESIAN_POINT('Ctrl Pts',(1.15530234155453,-0.407041111792943,1.25681160160691));
#3940=CARTESIAN_POINT('Ctrl Pts',(1.10126842659597,-0.387888272594439,1.30441816675528));
#3941=CARTESIAN_POINT('Ctrl Pts',(1.07446535104584,-0.373243761060364,1.32643091652006));
#3942=CARTESIAN_POINT('Ctrl Pts',(1.02199477007745,-0.335108247315848,1.36743459453896));
#3943=CARTESIAN_POINT('Ctrl Pts',(0.990027513266105,-0.303141259068211,
1.39055359345152));
#3944=CARTESIAN_POINT('Ctrl Pts',(0.940896403863071,-0.236152929235937,
1.42432715921571));
#3945=CARTESIAN_POINT('Ctrl Pts',(0.917859913453974,-0.192480977588835,
1.43904931717599));
#3946=CARTESIAN_POINT('Ctrl Pts',(0.895520212222106,-0.123823518623745,
1.45296717977858));
#3947=CARTESIAN_POINT('Ctrl Pts',(0.890059788636851,-0.101649918886749,
1.45630208793976));
#3948=CARTESIAN_POINT('Ctrl Pts',(0.886256117232622,-0.0793800000000001,
1.45861320581289));
#3949=CARTESIAN_POINT('Origin',(1.18440385848747,-0.07938,1.18440385848747));
#3950=CARTESIAN_POINT('Origin',(0.,-0.27783,0.));
#3951=CARTESIAN_POINT('',(0.404717578595295,-0.07938,1.65807299932179));
#3952=CARTESIAN_POINT('Origin',(0.,-0.07938,0.));
#3953=CARTESIAN_POINT('',(-0.404717578595296,-0.07938,1.65807299932179));
#3954=CARTESIAN_POINT('Ctrl Pts',(0.404717578595296,-0.0793800000000001,
1.65807299932179));
#3955=CARTESIAN_POINT('Ctrl Pts',(0.400393769631747,-0.101649918886749,
1.65912839404491));
#3956=CARTESIAN_POINT('Ctrl Pts',(0.394174530911058,-0.123823518623745,
1.66063136041479));
#3957=CARTESIAN_POINT('Ctrl Pts',(0.368536561654407,-0.192480977588835,
1.66658649961961));
#3958=CARTESIAN_POINT('Ctrl Pts',(0.341837165343982,-0.236152929235937,
1.67246562047521));
#3959=CARTESIAN_POINT('Ctrl Pts',(0.283214707341173,-0.303141259068211,
1.68332504372461));
#3960=CARTESIAN_POINT('Ctrl Pts',(0.244262842368623,-0.335108247315849,
1.68958170688653));
#3961=CARTESIAN_POINT('Ctrl Pts',(0.178166559972324,-0.373243761060364,
1.69769003172132));
#3962=CARTESIAN_POINT('Ctrl Pts',(0.143648558862931,-0.387888272594439,
1.70107730356824));
#3963=CARTESIAN_POINT('Ctrl Pts',(0.0717778861362652,-0.407041111792943,
1.70562212620408));
#3964=CARTESIAN_POINT('Ctrl Pts',(0.0344244045173309,-0.411552957311693,
1.706752));
#3965=CARTESIAN_POINT('Ctrl Pts',(-0.0344244045173315,-0.411552957311693,
1.706752));
#3966=CARTESIAN_POINT('Ctrl Pts',(-0.0717778861362658,-0.407041111792943,
1.70562212620408));
#3967=CARTESIAN_POINT('Ctrl Pts',(-0.143648558862932,-0.387888272594439,
1.70107730356824));
#3968=CARTESIAN_POINT('Ctrl Pts',(-0.178166559972325,-0.373243761060364,
1.69769003172132));
#3969=CARTESIAN_POINT('Ctrl Pts',(-0.244262842368624,-0.335108247315849,
1.68958170688653));
#3970=CARTESIAN_POINT('Ctrl Pts',(-0.283214707341173,-0.303141259068212,
1.68332504372461));
#3971=CARTESIAN_POINT('Ctrl Pts',(-0.341837165343982,-0.236152929235937,
1.67246562047521));
#3972=CARTESIAN_POINT('Ctrl Pts',(-0.368536561654408,-0.192480977588835,
1.66658649961961));
#3973=CARTESIAN_POINT('Ctrl Pts',(-0.394174530911059,-0.123823518623745,
1.66063136041479));
#3974=CARTESIAN_POINT('Ctrl Pts',(-0.400393769631748,-0.101649918886749,
1.65912839404491));
#3975=CARTESIAN_POINT('Ctrl Pts',(-0.404717578595297,-0.0793800000000001,
1.65807299932179));
#3976=CARTESIAN_POINT('',(-0.886256117232624,-0.07938,1.45861320581289));
#3977=CARTESIAN_POINT('Origin',(0.,-0.07938,0.));
#3978=CARTESIAN_POINT('',(-1.45861320581289,-0.07938,0.886256117232623));
#3979=CARTESIAN_POINT('Ctrl Pts',(-0.886256117232623,-0.0793800000000001,
1.45861320581289));
#3980=CARTESIAN_POINT('Ctrl Pts',(-0.890059788636852,-0.101649918886749,
1.45630208793976));
#3981=CARTESIAN_POINT('Ctrl Pts',(-0.895520212222106,-0.123823518623745,
1.45296717977858));
#3982=CARTESIAN_POINT('Ctrl Pts',(-0.917859913453974,-0.192480977588835,
1.43904931717599));
#3983=CARTESIAN_POINT('Ctrl Pts',(-0.940896403863071,-0.236152929235937,
1.4243271592157));
#3984=CARTESIAN_POINT('Ctrl Pts',(-0.990027513266105,-0.303141259068211,
1.39055359345152));
#3985=CARTESIAN_POINT('Ctrl Pts',(-1.02199477007745,-0.335108247315848,
1.36743459453896));
#3986=CARTESIAN_POINT('Ctrl Pts',(-1.07446535104584,-0.373243761060364,
1.32643091652006));
#3987=CARTESIAN_POINT('Ctrl Pts',(-1.10126842659597,-0.387888272594439,
1.30441816675528));
#3988=CARTESIAN_POINT('Ctrl Pts',(-1.15530234155453,-0.407041111792943,
1.25681160160691));
#3989=CARTESIAN_POINT('Ctrl Pts',(-1.18251418313119,-0.411552957311693,
1.23119764287622));
#3990=CARTESIAN_POINT('Ctrl Pts',(-1.23119764287622,-0.411552957311693,
1.18251418313119));
#3991=CARTESIAN_POINT('Ctrl Pts',(-1.25681160160691,-0.407041111792943,
1.15530234155453));
#3992=CARTESIAN_POINT('Ctrl Pts',(-1.30441816675528,-0.387888272594439,
1.10126842659597));
#3993=CARTESIAN_POINT('Ctrl Pts',(-1.32643091652006,-0.373243761060365,
1.07446535104584));
#3994=CARTESIAN_POINT('Ctrl Pts',(-1.36743459453896,-0.335108247315849,
1.02199477007745));
#3995=CARTESIAN_POINT('Ctrl Pts',(-1.39055359345152,-0.303141259068212,
0.990027513266106));
#3996=CARTESIAN_POINT('Ctrl Pts',(-1.4243271592157,-0.236152929235938,0.940896403863071));
#3997=CARTESIAN_POINT('Ctrl Pts',(-1.43904931717599,-0.192480977588836,
0.917859913453974));
#3998=CARTESIAN_POINT('Ctrl Pts',(-1.45296717977858,-0.123823518623746,
0.895520212222106));
#3999=CARTESIAN_POINT('Ctrl Pts',(-1.45630208793976,-0.101649918886749,
0.890059788636852));
#4000=CARTESIAN_POINT('Ctrl Pts',(-1.45861320581289,-0.0793800000000001,
0.886256117232623));
#4001=CARTESIAN_POINT('',(-1.65807299932179,-0.07938,0.404717578595295));
#4002=CARTESIAN_POINT('Origin',(0.,-0.07938,0.));
#4003=CARTESIAN_POINT('',(-1.706752,-0.411552957311693,2.08591827245526E-16));
#4004=CARTESIAN_POINT('Ctrl Pts',(-1.65807299932179,-0.0793800000000001,
0.404717578595296));
#4005=CARTESIAN_POINT('Ctrl Pts',(-1.65912839404491,-0.101649918886749,
0.400393769631747));
#4006=CARTESIAN_POINT('Ctrl Pts',(-1.66063136041479,-0.123823518623745,
0.394174530911058));
#4007=CARTESIAN_POINT('Ctrl Pts',(-1.66658649961961,-0.192480977588835,
0.368536561654407));
#4008=CARTESIAN_POINT('Ctrl Pts',(-1.67246562047521,-0.236152929235937,
0.341837165343982));
#4009=CARTESIAN_POINT('Ctrl Pts',(-1.68332504372461,-0.303141259068211,
0.283214707341173));
#4010=CARTESIAN_POINT('Ctrl Pts',(-1.68958170688653,-0.335108247315848,
0.244262842368623));
#4011=CARTESIAN_POINT('Ctrl Pts',(-1.69769003172132,-0.373243761060364,
0.178166559972324));
#4012=CARTESIAN_POINT('Ctrl Pts',(-1.70107730356824,-0.387888272594439,
0.143648558862931));
#4013=CARTESIAN_POINT('Ctrl Pts',(-1.70562212620408,-0.407041111792943,
0.0717778861362656));
#4014=CARTESIAN_POINT('Ctrl Pts',(-1.706752,-0.411552957311693,0.0344244045173313));
#4015=CARTESIAN_POINT('Ctrl Pts',(-1.706752,-0.411552957311693,2.08166817117217E-16));
#4016=CARTESIAN_POINT('',(-1.706752,-0.47628,2.09016837373834E-16));
#4017=CARTESIAN_POINT('',(-1.706752,-0.27783,2.09016837373834E-16));
#4018=CARTESIAN_POINT('Origin',(0.,-0.47628,0.));
#4019=CARTESIAN_POINT('',(-1.65807299932179,-0.07938,-0.404717578595296));
#4020=CARTESIAN_POINT('Ctrl Pts',(-1.706752,-0.411552957311693,2.0122792321331E-16));
#4021=CARTESIAN_POINT('Ctrl Pts',(-1.706752,-0.411552957311693,-0.0344244045173309));
#4022=CARTESIAN_POINT('Ctrl Pts',(-1.70562212620408,-0.407041111792943,
-0.0717778861362652));
#4023=CARTESIAN_POINT('Ctrl Pts',(-1.70107730356824,-0.387888272594439,
-0.143648558862931));
#4024=CARTESIAN_POINT('Ctrl Pts',(-1.69769003172132,-0.373243761060365,
-0.178166559972324));
#4025=CARTESIAN_POINT('Ctrl Pts',(-1.68958170688653,-0.335108247315849,
-0.244262842368623));
#4026=CARTESIAN_POINT('Ctrl Pts',(-1.68332504372461,-0.303141259068212,
-0.283214707341173));
#4027=CARTESIAN_POINT('Ctrl Pts',(-1.67246562047521,-0.236152929235938,
-0.341837165343982));
#4028=CARTESIAN_POINT('Ctrl Pts',(-1.66658649961961,-0.192480977588836,
-0.368536561654407));
#4029=CARTESIAN_POINT('Ctrl Pts',(-1.66063136041479,-0.123823518623745,
-0.394174530911059));
#4030=CARTESIAN_POINT('Ctrl Pts',(-1.65912839404491,-0.101649918886749,
-0.400393769631748));
#4031=CARTESIAN_POINT('Ctrl Pts',(-1.65807299932179,-0.0793800000000001,
-0.404717578595296));
#4032=CARTESIAN_POINT('',(-1.45861320581289,-0.07938,-0.886256117232623));
#4033=CARTESIAN_POINT('Origin',(0.,-0.07938,0.));
#4034=CARTESIAN_POINT('',(-0.886256117232623,-0.07938,-1.45861320581289));
#4035=CARTESIAN_POINT('Ctrl Pts',(-1.45861320581289,-0.0793800000000001,
-0.886256117232623));
#4036=CARTESIAN_POINT('Ctrl Pts',(-1.45630208793976,-0.101649918886749,
-0.890059788636852));
#4037=CARTESIAN_POINT('Ctrl Pts',(-1.45296717977858,-0.123823518623745,
-0.895520212222106));
#4038=CARTESIAN_POINT('Ctrl Pts',(-1.43904931717599,-0.192480977588835,
-0.917859913453974));
#4039=CARTESIAN_POINT('Ctrl Pts',(-1.4243271592157,-0.236152929235937,-0.940896403863072));
#4040=CARTESIAN_POINT('Ctrl Pts',(-1.39055359345152,-0.303141259068212,
-0.990027513266106));
#4041=CARTESIAN_POINT('Ctrl Pts',(-1.36743459453896,-0.335108247315849,
-1.02199477007745));
#4042=CARTESIAN_POINT('Ctrl Pts',(-1.32643091652006,-0.373243761060364,
-1.07446535104584));
#4043=CARTESIAN_POINT('Ctrl Pts',(-1.30441816675528,-0.387888272594439,
-1.10126842659597));
#4044=CARTESIAN_POINT('Ctrl Pts',(-1.25681160160691,-0.407041111792943,
-1.15530234155453));
#4045=CARTESIAN_POINT('Ctrl Pts',(-1.23119764287622,-0.411552957311693,
-1.18251418313119));
#4046=CARTESIAN_POINT('Ctrl Pts',(-1.18251418313119,-0.411552957311693,
-1.23119764287622));
#4047=CARTESIAN_POINT('Ctrl Pts',(-1.15530234155453,-0.407041111792943,
-1.25681160160691));
#4048=CARTESIAN_POINT('Ctrl Pts',(-1.10126842659597,-0.387888272594439,
-1.30441816675528));
#4049=CARTESIAN_POINT('Ctrl Pts',(-1.07446535104584,-0.373243761060364,
-1.32643091652006));
#4050=CARTESIAN_POINT('Ctrl Pts',(-1.02199477007745,-0.335108247315848,
-1.36743459453896));
#4051=CARTESIAN_POINT('Ctrl Pts',(-0.990027513266105,-0.303141259068211,
-1.39055359345152));
#4052=CARTESIAN_POINT('Ctrl Pts',(-0.940896403863071,-0.236152929235936,
-1.42432715921571));
#4053=CARTESIAN_POINT('Ctrl Pts',(-0.917859913453974,-0.192480977588835,
-1.43904931717599));
#4054=CARTESIAN_POINT('Ctrl Pts',(-0.895520212222106,-0.123823518623745,
-1.45296717977858));
#4055=CARTESIAN_POINT('Ctrl Pts',(-0.890059788636851,-0.101649918886749,
-1.45630208793976));
#4056=CARTESIAN_POINT('Ctrl Pts',(-0.886256117232623,-0.0793800000000001,
-1.45861320581289));
#4057=CARTESIAN_POINT('',(-0.404717578595295,-0.07938,-1.65807299932179));
#4058=CARTESIAN_POINT('Origin',(0.,-0.07938,0.));
#4059=CARTESIAN_POINT('',(0.404717578595296,-0.07938,-1.65807299932179));
#4060=CARTESIAN_POINT('Ctrl Pts',(-0.404717578595296,-0.0793800000000001,
-1.65807299932179));
#4061=CARTESIAN_POINT('Ctrl Pts',(-0.400393769631747,-0.101649918886749,
-1.65912839404491));
#4062=CARTESIAN_POINT('Ctrl Pts',(-0.394174530911058,-0.123823518623746,
-1.66063136041479));
#4063=CARTESIAN_POINT('Ctrl Pts',(-0.368536561654407,-0.192480977588836,
-1.66658649961961));
#4064=CARTESIAN_POINT('Ctrl Pts',(-0.341837165343982,-0.236152929235938,
-1.67246562047521));
#4065=CARTESIAN_POINT('Ctrl Pts',(-0.283214707341173,-0.303141259068212,
-1.68332504372461));
#4066=CARTESIAN_POINT('Ctrl Pts',(-0.244262842368623,-0.335108247315849,
-1.68958170688653));
#4067=CARTESIAN_POINT('Ctrl Pts',(-0.178166559972324,-0.373243761060364,
-1.69769003172132));
#4068=CARTESIAN_POINT('Ctrl Pts',(-0.143648558862931,-0.387888272594439,
-1.70107730356824));
#4069=CARTESIAN_POINT('Ctrl Pts',(-0.0717778861362653,-0.407041111792943,
-1.70562212620408));
#4070=CARTESIAN_POINT('Ctrl Pts',(-0.034424404517331,-0.411552957311693,
-1.706752));
#4071=CARTESIAN_POINT('Ctrl Pts',(0.0344244045173312,-0.411552957311693,
-1.706752));
#4072=CARTESIAN_POINT('Ctrl Pts',(0.0717778861362655,-0.407041111792943,
-1.70562212620408));
#4073=CARTESIAN_POINT('Ctrl Pts',(0.143648558862931,-0.387888272594439,
-1.70107730356824));
#4074=CARTESIAN_POINT('Ctrl Pts',(0.178166559972324,-0.373243761060364,
-1.69769003172132));
#4075=CARTESIAN_POINT('Ctrl Pts',(0.244262842368623,-0.335108247315849,
-1.68958170688653));
#4076=CARTESIAN_POINT('Ctrl Pts',(0.283214707341173,-0.303141259068212,
-1.68332504372461));
#4077=CARTESIAN_POINT('Ctrl Pts',(0.341837165343982,-0.236152929235937,
-1.67246562047521));
#4078=CARTESIAN_POINT('Ctrl Pts',(0.368536561654407,-0.192480977588835,
-1.66658649961961));
#4079=CARTESIAN_POINT('Ctrl Pts',(0.394174530911059,-0.123823518623745,
-1.66063136041479));
#4080=CARTESIAN_POINT('Ctrl Pts',(0.400393769631748,-0.101649918886749,
-1.65912839404491));
#4081=CARTESIAN_POINT('Ctrl Pts',(0.404717578595296,-0.0793800000000001,
-1.65807299932179));
#4082=CARTESIAN_POINT('',(0.886256117232623,-0.07938,-1.45861320581289));
#4083=CARTESIAN_POINT('Origin',(0.,-0.07938,0.));
#4084=CARTESIAN_POINT('',(1.45861320581289,-0.07938,-0.886256117232623));
#4085=CARTESIAN_POINT('Ctrl Pts',(0.886256117232623,-0.0793800000000001,
-1.45861320581289));
#4086=CARTESIAN_POINT('Ctrl Pts',(0.890059788636852,-0.101649918886749,
-1.45630208793976));
#4087=CARTESIAN_POINT('Ctrl Pts',(0.895520212222106,-0.123823518623745,
-1.45296717977858));
#4088=CARTESIAN_POINT('Ctrl Pts',(0.917859913453974,-0.192480977588835,
-1.43904931717599));
#4089=CARTESIAN_POINT('Ctrl Pts',(0.940896403863072,-0.236152929235937,
-1.4243271592157));
#4090=CARTESIAN_POINT('Ctrl Pts',(0.990027513266106,-0.303141259068211,
-1.39055359345152));
#4091=CARTESIAN_POINT('Ctrl Pts',(1.02199477007745,-0.335108247315849,-1.36743459453896));
#4092=CARTESIAN_POINT('Ctrl Pts',(1.07446535104584,-0.373243761060364,-1.32643091652006));
#4093=CARTESIAN_POINT('Ctrl Pts',(1.10126842659597,-0.387888272594439,-1.30441816675528));
#4094=CARTESIAN_POINT('Ctrl Pts',(1.15530234155453,-0.407041111792943,-1.25681160160691));
#4095=CARTESIAN_POINT('Ctrl Pts',(1.18251418313119,-0.411552957311693,-1.23119764287622));
#4096=CARTESIAN_POINT('Ctrl Pts',(1.23119764287622,-0.411552957311693,-1.18251418313119));
#4097=CARTESIAN_POINT('Ctrl Pts',(1.25681160160691,-0.407041111792943,-1.15530234155453));
#4098=CARTESIAN_POINT('Ctrl Pts',(1.30441816675528,-0.387888272594439,-1.10126842659597));
#4099=CARTESIAN_POINT('Ctrl Pts',(1.32643091652006,-0.373243761060364,-1.07446535104584));
#4100=CARTESIAN_POINT('Ctrl Pts',(1.36743459453896,-0.335108247315849,-1.02199477007745));
#4101=CARTESIAN_POINT('Ctrl Pts',(1.39055359345152,-0.303141259068212,-0.990027513266105));
#4102=CARTESIAN_POINT('Ctrl Pts',(1.4243271592157,-0.236152929235937,-0.940896403863071));
#4103=CARTESIAN_POINT('Ctrl Pts',(1.43904931717599,-0.192480977588835,-0.917859913453974));
#4104=CARTESIAN_POINT('Ctrl Pts',(1.45296717977858,-0.123823518623745,-0.895520212222106));
#4105=CARTESIAN_POINT('Ctrl Pts',(1.45630208793976,-0.101649918886749,-0.890059788636852));
#4106=CARTESIAN_POINT('Ctrl Pts',(1.45861320581289,-0.0793800000000001,
-0.886256117232623));
#4107=CARTESIAN_POINT('',(1.65807299932179,-0.07938,-0.404717578595296));
#4108=CARTESIAN_POINT('Origin',(0.,-0.07938,0.));
#4109=CARTESIAN_POINT('',(1.65807299932179,-0.07938,0.404717578595296));
#4110=CARTESIAN_POINT('Ctrl Pts',(1.65807299932179,-0.0793800000000001,
-0.404717578595296));
#4111=CARTESIAN_POINT('Ctrl Pts',(1.65912839404491,-0.101649918886749,-0.400393769631747));
#4112=CARTESIAN_POINT('Ctrl Pts',(1.66063136041479,-0.123823518623745,-0.394174530911058));
#4113=CARTESIAN_POINT('Ctrl Pts',(1.66658649961961,-0.192480977588835,-0.368536561654407));
#4114=CARTESIAN_POINT('Ctrl Pts',(1.67246562047521,-0.236152929235937,-0.341837165343982));
#4115=CARTESIAN_POINT('Ctrl Pts',(1.68332504372461,-0.303141259068212,-0.283214707341173));
#4116=CARTESIAN_POINT('Ctrl Pts',(1.68958170688653,-0.335108247315849,-0.244262842368623));
#4117=CARTESIAN_POINT('Ctrl Pts',(1.69769003172132,-0.373243761060364,-0.178166559972324));
#4118=CARTESIAN_POINT('Ctrl Pts',(1.70107730356824,-0.387888272594439,-0.143648558862931));
#4119=CARTESIAN_POINT('Ctrl Pts',(1.70562212620408,-0.407041111792943,-0.0717778861362655));
#4120=CARTESIAN_POINT('Ctrl Pts',(1.706752,-0.411552957311693,-0.0344244045173312));
#4121=CARTESIAN_POINT('Ctrl Pts',(1.706752,-0.411552957311693,0.0344244045173312));
#4122=CARTESIAN_POINT('Ctrl Pts',(1.70562212620408,-0.407041111792943,0.0717778861362655));
#4123=CARTESIAN_POINT('Ctrl Pts',(1.70107730356824,-0.387888272594439,0.143648558862931));
#4124=CARTESIAN_POINT('Ctrl Pts',(1.69769003172132,-0.373243761060364,0.178166559972324));
#4125=CARTESIAN_POINT('Ctrl Pts',(1.68958170688653,-0.335108247315849,0.244262842368623));
#4126=CARTESIAN_POINT('Ctrl Pts',(1.68332504372461,-0.303141259068212,0.283214707341173));
#4127=CARTESIAN_POINT('Ctrl Pts',(1.67246562047521,-0.236152929235937,0.341837165343982));
#4128=CARTESIAN_POINT('Ctrl Pts',(1.66658649961961,-0.192480977588835,0.368536561654407));
#4129=CARTESIAN_POINT('Ctrl Pts',(1.66063136041479,-0.123823518623745,0.394174530911058));
#4130=CARTESIAN_POINT('Ctrl Pts',(1.65912839404491,-0.101649918886749,0.400393769631747));
#4131=CARTESIAN_POINT('Ctrl Pts',(1.65807299932179,-0.0793800000000001,
0.404717578595296));
#4132=CARTESIAN_POINT('Origin',(0.,-0.07938,0.));
#4133=CARTESIAN_POINT('Origin',(0.,-0.07938,0.));
#4134=CARTESIAN_POINT('',(0.397005914195118,-0.07938,1.59456899932179));
#4135=CARTESIAN_POINT('Origin',(0.,-0.07938,0.));
#4136=CARTESIAN_POINT('Origin',(-3.33066907387547E-16,-0.07938,1.675));
#4137=CARTESIAN_POINT('Origin',(-3.33066907387547E-16,0.,1.675));
#4138=CARTESIAN_POINT('',(-0.397005914195118,-0.07938,1.59456899932179));
#4139=CARTESIAN_POINT('Ctrl Pts',(-0.397005914195119,-0.0793800000000001,
1.59456899932179));
#4140=CARTESIAN_POINT('Ctrl Pts',(-0.3886265584581,-0.123401821157026,1.59665523941937));
#4141=CARTESIAN_POINT('Ctrl Pts',(-0.373030350867485,-0.166543350814306,
1.60050712143809));
#4142=CARTESIAN_POINT('Ctrl Pts',(-0.333298652394954,-0.237231147975234,
1.60919314384089));
#4143=CARTESIAN_POINT('Ctrl Pts',(-0.311480544243687,-0.266264900654909,
1.61365775139403));
#4144=CARTESIAN_POINT('Ctrl Pts',(-0.261368388670537,-0.317195968905306,
1.62252828437015));
#4145=CARTESIAN_POINT('Ctrl Pts',(-0.233069203882014,-0.33909093068465,
1.62691869420078));
#4146=CARTESIAN_POINT('Ctrl Pts',(-0.174042761838764,-0.373586846396559,
1.63426473152765));
#4147=CARTESIAN_POINT('Ctrl Pts',(-0.14036578147155,-0.388086240756494,
1.63761964365402));
#4148=CARTESIAN_POINT('Ctrl Pts',(-0.0701778381840615,-0.407068917407805,
1.64212536811722));
#4149=CARTESIAN_POINT('Ctrl Pts',(-0.0336652739555918,-0.411552957311693,
1.643248));
#4150=CARTESIAN_POINT('Ctrl Pts',(0.0336652739555913,-0.411552957311693,
1.643248));
#4151=CARTESIAN_POINT('Ctrl Pts',(0.070177838184061,-0.407068917407805,
1.64212536811722));
#4152=CARTESIAN_POINT('Ctrl Pts',(0.140365781471549,-0.388086240756494,
1.63761964365402));
#4153=CARTESIAN_POINT('Ctrl Pts',(0.174042761838763,-0.373586846396559,
1.63426473152765));
#4154=CARTESIAN_POINT('Ctrl Pts',(0.233069203882014,-0.33909093068465,1.62691869420078));
#4155=CARTESIAN_POINT('Ctrl Pts',(0.261368388670536,-0.317195968905306,
1.62252828437015));
#4156=CARTESIAN_POINT('Ctrl Pts',(0.311480544243686,-0.266264900654908,
1.61365775139403));
#4157=CARTESIAN_POINT('Ctrl Pts',(0.333298652394954,-0.237231147975234,
1.60919314384089));
#4158=CARTESIAN_POINT('Ctrl Pts',(0.373030350867484,-0.166543350814306,
1.60050712143809));
#4159=CARTESIAN_POINT('Ctrl Pts',(0.388626558458099,-0.123401821157026,
1.59665523941937));
#4160=CARTESIAN_POINT('Ctrl Pts',(0.397005914195118,-0.07938,1.59456899932179));
#4161=CARTESIAN_POINT('Origin',(-3.33066907387547E-16,-0.07938,1.675));
#4162=CARTESIAN_POINT('Origin',(0.,-0.07938,0.));
#4163=CARTESIAN_POINT('',(-0.846804978391754,-0.07938,1.40825612658882));
#4164=CARTESIAN_POINT('Origin',(0.,-0.07938,0.));
#4165=CARTESIAN_POINT('Origin',(-1.18440385848747,-0.07938,1.18440385848747));
#4166=CARTESIAN_POINT('Origin',(-1.18440385848747,0.,1.18440385848747));
#4167=CARTESIAN_POINT('',(-1.40825612658882,-0.07938,0.846804978391753));
#4168=CARTESIAN_POINT('Ctrl Pts',(-1.40825612658882,-0.0793800000000001,
0.846804978391753));
#4169=CARTESIAN_POINT('Ctrl Pts',(-1.40380622184538,-0.123401821157026,
0.854205272175555));
#4170=CARTESIAN_POINT('Ctrl Pts',(-1.39550172959303,-0.166543350814306,
0.867957148219442));
#4171=CARTESIAN_POINT('Ctrl Pts',(-1.3735491215176,-0.237231147975235,0.902193646979983));
#4172=CARTESIAN_POINT('Ctrl Pts',(-1.36127834356734,-0.266264900654909,
0.920778333482565));
#4173=CARTESIAN_POINT('Ctrl Pts',(-1.33211611256184,-0.317195968905306,
0.962485392528369));
#4174=CARTESIAN_POINT('Ctrl Pts',(-1.31521005565926,-0.339090930684651,
0.985600426557816));
#4175=CARTESIAN_POINT('Ctrl Pts',(-1.27866649102984,-0.373586846396559,
1.03253285680459));
#4176=CARTESIAN_POINT('Ctrl Pts',(-1.25722555095714,-0.388086240756494,
1.05871835910697));
#4177=CARTESIAN_POINT('Ctrl Pts',(-1.2107812086231,-0.407068917407805,1.11153475808518));
#4178=CARTESIAN_POINT('Ctrl Pts',(-1.18575674747573,-0.411552957311693,
1.13814686046673));
#4179=CARTESIAN_POINT('Ctrl Pts',(-1.13814686046673,-0.411552957311693,
1.18575674747573));
#4180=CARTESIAN_POINT('Ctrl Pts',(-1.11153475808518,-0.407068917407805,
1.2107812086231));
#4181=CARTESIAN_POINT('Ctrl Pts',(-1.05871835910697,-0.388086240756494,
1.25722555095714));
#4182=CARTESIAN_POINT('Ctrl Pts',(-1.03253285680459,-0.373586846396559,
1.27866649102984));
#4183=CARTESIAN_POINT('Ctrl Pts',(-0.985600426557816,-0.33909093068465,
1.31521005565926));
#4184=CARTESIAN_POINT('Ctrl Pts',(-0.962485392528369,-0.317195968905306,
1.33211611256184));
#4185=CARTESIAN_POINT('Ctrl Pts',(-0.920778333482565,-0.266264900654908,
1.36127834356734));
#4186=CARTESIAN_POINT('Ctrl Pts',(-0.902193646979983,-0.237231147975234,
1.3735491215176));
#4187=CARTESIAN_POINT('Ctrl Pts',(-0.867957148219442,-0.166543350814306,
1.39550172959303));
#4188=CARTESIAN_POINT('Ctrl Pts',(-0.854205272175555,-0.123401821157026,
1.40380622184538));
#4189=CARTESIAN_POINT('Ctrl Pts',(-0.846804978391753,-0.0793800000000001,
1.40825612658882));
#4190=CARTESIAN_POINT('Origin',(-1.18440385848747,-0.07938,1.18440385848747));
#4191=CARTESIAN_POINT('Origin',(0.,-0.07938,0.));
#4192=CARTESIAN_POINT('',(-1.59456899932179,-0.07938,0.397005914195118));
#4193=CARTESIAN_POINT('Origin',(0.,-0.07938,0.));
#4194=CARTESIAN_POINT('Origin',(-1.675,-0.07938,-2.22044604925031E-16));
#4195=CARTESIAN_POINT('Origin',(-1.675,0.,-2.22044604925031E-16));
#4196=CARTESIAN_POINT('',(-1.59456899932179,-0.07938,-0.397005914195118));
#4197=CARTESIAN_POINT('',(-1.643248,-0.411552957311693,3.47540551556327E-18));
#4198=CARTESIAN_POINT('Ctrl Pts',(-1.59456899932179,-0.0793800000000001,
-0.397005914195119));
#4199=CARTESIAN_POINT('Ctrl Pts',(-1.59665523941937,-0.123401821157026,
-0.388626558458099));
#4200=CARTESIAN_POINT('Ctrl Pts',(-1.60050712143809,-0.166543350814306,
-0.373030350867485));
#4201=CARTESIAN_POINT('Ctrl Pts',(-1.60919314384089,-0.237231147975234,
-0.333298652394954));
#4202=CARTESIAN_POINT('Ctrl Pts',(-1.61365775139403,-0.266264900654909,
-0.311480544243686));
#4203=CARTESIAN_POINT('Ctrl Pts',(-1.62252828437015,-0.317195968905306,
-0.261368388670537));
#4204=CARTESIAN_POINT('Ctrl Pts',(-1.62691869420078,-0.33909093068465,-0.233069203882014));
#4205=CARTESIAN_POINT('Ctrl Pts',(-1.63426473152765,-0.373586846396559,
-0.174042761838764));
#4206=CARTESIAN_POINT('Ctrl Pts',(-1.63761964365402,-0.388086240756494,
-0.140365781471549));
#4207=CARTESIAN_POINT('Ctrl Pts',(-1.64212536811722,-0.407068917407805,
-0.0701778381840614));
#4208=CARTESIAN_POINT('Ctrl Pts',(-1.643248,-0.411552957311693,-0.0336652739555917));
#4209=CARTESIAN_POINT('Ctrl Pts',(-1.643248,-0.411552957311693,-2.0122792321331E-16));
#4210=CARTESIAN_POINT('Origin',(-1.675,-0.07938,-2.22044604925031E-16));
#4211=CARTESIAN_POINT('Ctrl Pts',(-1.643248,-0.411552957311693,-1.94289029309402E-16));
#4212=CARTESIAN_POINT('Ctrl Pts',(-1.643248,-0.411552957311693,0.0336652739555913));
#4213=CARTESIAN_POINT('Ctrl Pts',(-1.64212536811722,-0.407068917407805,
0.0701778381840609));
#4214=CARTESIAN_POINT('Ctrl Pts',(-1.63761964365402,-0.388086240756494,
0.140365781471549));
#4215=CARTESIAN_POINT('Ctrl Pts',(-1.63426473152765,-0.373586846396559,
0.174042761838763));
#4216=CARTESIAN_POINT('Ctrl Pts',(-1.62691869420078,-0.33909093068465,0.233069203882014));
#4217=CARTESIAN_POINT('Ctrl Pts',(-1.62252828437015,-0.317195968905306,
0.261368388670536));
#4218=CARTESIAN_POINT('Ctrl Pts',(-1.61365775139403,-0.266264900654909,
0.311480544243686));
#4219=CARTESIAN_POINT('Ctrl Pts',(-1.60919314384089,-0.237231147975235,
0.333298652394954));
#4220=CARTESIAN_POINT('Ctrl Pts',(-1.60050712143809,-0.166543350814306,
0.373030350867484));
#4221=CARTESIAN_POINT('Ctrl Pts',(-1.59665523941937,-0.123401821157026,
0.388626558458099));
#4222=CARTESIAN_POINT('Ctrl Pts',(-1.59456899932179,-0.0793800000000001,
0.397005914195118));
#4223=CARTESIAN_POINT('Origin',(0.,-0.07938,0.));
#4224=CARTESIAN_POINT('',(-1.40825612658882,-0.07938,-0.846804978391753));
#4225=CARTESIAN_POINT('Origin',(0.,-0.07938,0.));
#4226=CARTESIAN_POINT('Origin',(-1.18440385848747,-0.07938,-1.18440385848747));
#4227=CARTESIAN_POINT('Origin',(-1.18440385848747,0.,-1.18440385848747));
#4228=CARTESIAN_POINT('',(-0.846804978391753,-0.07938,-1.40825612658882));
#4229=CARTESIAN_POINT('Ctrl Pts',(-0.846804978391753,-0.0793800000000001,
-1.40825612658882));
#4230=CARTESIAN_POINT('Ctrl Pts',(-0.854205272175555,-0.123401821157026,
-1.40380622184538));
#4231=CARTESIAN_POINT('Ctrl Pts',(-0.867957148219442,-0.166543350814306,
-1.39550172959303));
#4232=CARTESIAN_POINT('Ctrl Pts',(-0.902193646979982,-0.237231147975234,
-1.3735491215176));
#4233=CARTESIAN_POINT('Ctrl Pts',(-0.920778333482564,-0.266264900654908,
-1.36127834356734));
#4234=CARTESIAN_POINT('Ctrl Pts',(-0.962485392528368,-0.317195968905306,
-1.33211611256184));
#4235=CARTESIAN_POINT('Ctrl Pts',(-0.985600426557816,-0.33909093068465,
-1.31521005565926));
#4236=CARTESIAN_POINT('Ctrl Pts',(-1.03253285680459,-0.373586846396559,
-1.27866649102984));
#4237=CARTESIAN_POINT('Ctrl Pts',(-1.05871835910697,-0.388086240756494,
-1.25722555095714));
#4238=CARTESIAN_POINT('Ctrl Pts',(-1.11153475808518,-0.407068917407805,
-1.2107812086231));
#4239=CARTESIAN_POINT('Ctrl Pts',(-1.13814686046673,-0.411552957311693,
-1.18575674747573));
#4240=CARTESIAN_POINT('Ctrl Pts',(-1.18575674747573,-0.411552957311693,
-1.13814686046673));
#4241=CARTESIAN_POINT('Ctrl Pts',(-1.2107812086231,-0.407068917407805,-1.11153475808518));
#4242=CARTESIAN_POINT('Ctrl Pts',(-1.25722555095714,-0.388086240756494,
-1.05871835910697));
#4243=CARTESIAN_POINT('Ctrl Pts',(-1.27866649102984,-0.373586846396559,
-1.03253285680459));
#4244=CARTESIAN_POINT('Ctrl Pts',(-1.31521005565926,-0.33909093068465,-0.985600426557816));
#4245=CARTESIAN_POINT('Ctrl Pts',(-1.33211611256184,-0.317195968905306,
-0.962485392528369));
#4246=CARTESIAN_POINT('Ctrl Pts',(-1.36127834356734,-0.266264900654909,
-0.920778333482565));
#4247=CARTESIAN_POINT('Ctrl Pts',(-1.3735491215176,-0.237231147975234,-0.902193646979983));
#4248=CARTESIAN_POINT('Ctrl Pts',(-1.39550172959303,-0.166543350814306,
-0.867957148219442));
#4249=CARTESIAN_POINT('Ctrl Pts',(-1.40380622184538,-0.123401821157026,
-0.854205272175555));
#4250=CARTESIAN_POINT('Ctrl Pts',(-1.40825612658882,-0.07938,-0.846804978391753));
#4251=CARTESIAN_POINT('Origin',(-1.18440385848747,-0.07938,-1.18440385848747));
#4252=CARTESIAN_POINT('Origin',(0.,-0.07938,0.));
#4253=CARTESIAN_POINT('',(-0.397005914195118,-0.07938,-1.59456899932179));
#4254=CARTESIAN_POINT('Origin',(0.,-0.07938,0.));
#4255=CARTESIAN_POINT('Origin',(1.11022302462516E-16,-0.07938,-1.675));
#4256=CARTESIAN_POINT('Origin',(1.11022302462516E-16,0.,-1.675));
#4257=CARTESIAN_POINT('',(0.397005914195118,-0.07938,-1.59456899932179));
#4258=CARTESIAN_POINT('Ctrl Pts',(0.397005914195119,-0.0793800000000001,
-1.59456899932179));
#4259=CARTESIAN_POINT('Ctrl Pts',(0.388626558458099,-0.123401821157026,
-1.59665523941937));
#4260=CARTESIAN_POINT('Ctrl Pts',(0.373030350867485,-0.166543350814306,
-1.60050712143809));
#4261=CARTESIAN_POINT('Ctrl Pts',(0.333298652394954,-0.237231147975234,
-1.60919314384089));
#4262=CARTESIAN_POINT('Ctrl Pts',(0.311480544243686,-0.266264900654909,
-1.61365775139403));
#4263=CARTESIAN_POINT('Ctrl Pts',(0.261368388670537,-0.317195968905306,
-1.62252828437015));
#4264=CARTESIAN_POINT('Ctrl Pts',(0.233069203882014,-0.33909093068465,-1.62691869420078));
#4265=CARTESIAN_POINT('Ctrl Pts',(0.174042761838763,-0.373586846396559,
-1.63426473152765));
#4266=CARTESIAN_POINT('Ctrl Pts',(0.140365781471549,-0.388086240756494,
-1.63761964365402));
#4267=CARTESIAN_POINT('Ctrl Pts',(0.0701778381840612,-0.407068917407805,
-1.64212536811722));
#4268=CARTESIAN_POINT('Ctrl Pts',(0.0336652739555916,-0.411552957311693,
-1.643248));
#4269=CARTESIAN_POINT('Ctrl Pts',(-0.0336652739555915,-0.411552957311693,
-1.643248));
#4270=CARTESIAN_POINT('Ctrl Pts',(-0.0701778381840612,-0.407068917407805,
-1.64212536811722));
#4271=CARTESIAN_POINT('Ctrl Pts',(-0.140365781471549,-0.388086240756494,
-1.63761964365402));
#4272=CARTESIAN_POINT('Ctrl Pts',(-0.174042761838764,-0.373586846396559,
-1.63426473152765));
#4273=CARTESIAN_POINT('Ctrl Pts',(-0.233069203882014,-0.33909093068465,
-1.62691869420078));
#4274=CARTESIAN_POINT('Ctrl Pts',(-0.261368388670536,-0.317195968905306,
-1.62252828437015));
#4275=CARTESIAN_POINT('Ctrl Pts',(-0.311480544243686,-0.266264900654908,
-1.61365775139403));
#4276=CARTESIAN_POINT('Ctrl Pts',(-0.333298652394954,-0.237231147975234,
-1.60919314384089));
#4277=CARTESIAN_POINT('Ctrl Pts',(-0.373030350867485,-0.166543350814306,
-1.60050712143809));
#4278=CARTESIAN_POINT('Ctrl Pts',(-0.388626558458099,-0.123401821157026,
-1.59665523941937));
#4279=CARTESIAN_POINT('Ctrl Pts',(-0.397005914195118,-0.07938,-1.59456899932179));
#4280=CARTESIAN_POINT('Origin',(1.11022302462516E-16,-0.07938,-1.675));
#4281=CARTESIAN_POINT('Origin',(0.,-0.07938,0.));
#4282=CARTESIAN_POINT('',(0.846804978391753,-0.07938,-1.40825612658882));
#4283=CARTESIAN_POINT('Origin',(0.,-0.07938,0.));
#4284=CARTESIAN_POINT('Origin',(1.18440385848747,-0.07938,-1.18440385848747));
#4285=CARTESIAN_POINT('Origin',(1.18440385848747,0.,-1.18440385848747));
#4286=CARTESIAN_POINT('',(1.40825612658882,-0.07938,-0.846804978391753));
#4287=CARTESIAN_POINT('Ctrl Pts',(1.40825612658882,-0.0793800000000001,
-0.846804978391753));
#4288=CARTESIAN_POINT('Ctrl Pts',(1.40380622184538,-0.123401821157026,-0.854205272175555));
#4289=CARTESIAN_POINT('Ctrl Pts',(1.39550172959303,-0.166543350814306,-0.867957148219442));
#4290=CARTESIAN_POINT('Ctrl Pts',(1.3735491215176,-0.237231147975234,-0.902193646979983));
#4291=CARTESIAN_POINT('Ctrl Pts',(1.36127834356734,-0.266264900654908,-0.920778333482565));
#4292=CARTESIAN_POINT('Ctrl Pts',(1.33211611256184,-0.317195968905306,-0.962485392528369));
#4293=CARTESIAN_POINT('Ctrl Pts',(1.31521005565926,-0.33909093068465,-0.985600426557816));
#4294=CARTESIAN_POINT('Ctrl Pts',(1.27866649102984,-0.373586846396559,-1.03253285680459));
#4295=CARTESIAN_POINT('Ctrl Pts',(1.25722555095714,-0.388086240756494,-1.05871835910697));
#4296=CARTESIAN_POINT('Ctrl Pts',(1.2107812086231,-0.407068917407805,-1.11153475808518));
#4297=CARTESIAN_POINT('Ctrl Pts',(1.18575674747573,-0.411552957311693,-1.13814686046673));
#4298=CARTESIAN_POINT('Ctrl Pts',(1.13814686046673,-0.411552957311693,-1.18575674747573));
#4299=CARTESIAN_POINT('Ctrl Pts',(1.11153475808518,-0.407068917407805,-1.2107812086231));
#4300=CARTESIAN_POINT('Ctrl Pts',(1.05871835910697,-0.388086240756494,-1.25722555095714));
#4301=CARTESIAN_POINT('Ctrl Pts',(1.03253285680459,-0.373586846396559,-1.27866649102984));
#4302=CARTESIAN_POINT('Ctrl Pts',(0.985600426557816,-0.33909093068465,-1.31521005565926));
#4303=CARTESIAN_POINT('Ctrl Pts',(0.962485392528369,-0.317195968905306,
-1.33211611256184));
#4304=CARTESIAN_POINT('Ctrl Pts',(0.920778333482565,-0.266264900654909,
-1.36127834356734));
#4305=CARTESIAN_POINT('Ctrl Pts',(0.902193646979983,-0.237231147975234,
-1.3735491215176));
#4306=CARTESIAN_POINT('Ctrl Pts',(0.867957148219442,-0.166543350814306,
-1.39550172959303));
#4307=CARTESIAN_POINT('Ctrl Pts',(0.854205272175555,-0.123401821157026,
-1.40380622184538));
#4308=CARTESIAN_POINT('Ctrl Pts',(0.846804978391753,-0.0793800000000001,
-1.40825612658882));
#4309=CARTESIAN_POINT('Origin',(1.18440385848747,-0.07938,-1.18440385848747));
#4310=CARTESIAN_POINT('Origin',(0.,-0.27783,0.));
#4311=CARTESIAN_POINT('',(-1.643248,-0.47628,2.01239840340529E-16));
#4312=CARTESIAN_POINT('Origin',(0.,-0.47628,0.));
#4313=CARTESIAN_POINT('',(-1.643248,-0.27783,2.01239840340529E-16));
#4314=CARTESIAN_POINT('',(1.59456899932179,-0.07938,0.397005914195118));
#4315=CARTESIAN_POINT('Origin',(0.,-0.07938,0.));
#4316=CARTESIAN_POINT('',(1.59456899932179,-0.07938,-0.397005914195118));
#4317=CARTESIAN_POINT('Ctrl Pts',(1.59456899932179,-0.0793800000000001,
0.397005914195118));
#4318=CARTESIAN_POINT('Ctrl Pts',(1.59665523941937,-0.123401821157026,0.388626558458099));
#4319=CARTESIAN_POINT('Ctrl Pts',(1.60050712143809,-0.166543350814306,0.373030350867485));
#4320=CARTESIAN_POINT('Ctrl Pts',(1.60919314384089,-0.237231147975234,0.333298652394954));
#4321=CARTESIAN_POINT('Ctrl Pts',(1.61365775139403,-0.266264900654909,0.311480544243686));
#4322=CARTESIAN_POINT('Ctrl Pts',(1.62252828437015,-0.317195968905306,0.261368388670537));
#4323=CARTESIAN_POINT('Ctrl Pts',(1.62691869420078,-0.33909093068465,0.233069203882014));
#4324=CARTESIAN_POINT('Ctrl Pts',(1.63426473152765,-0.373586846396559,0.174042761838764));
#4325=CARTESIAN_POINT('Ctrl Pts',(1.63761964365402,-0.388086240756494,0.140365781471549));
#4326=CARTESIAN_POINT('Ctrl Pts',(1.64212536811722,-0.407068917407805,0.0701778381840612));
#4327=CARTESIAN_POINT('Ctrl Pts',(1.643248,-0.411552957311693,0.0336652739555916));
#4328=CARTESIAN_POINT('Ctrl Pts',(1.643248,-0.411552957311693,-0.0336652739555916));
#4329=CARTESIAN_POINT('Ctrl Pts',(1.64212536811722,-0.407068917407805,-0.0701778381840612));
#4330=CARTESIAN_POINT('Ctrl Pts',(1.63761964365402,-0.388086240756494,-0.140365781471549));
#4331=CARTESIAN_POINT('Ctrl Pts',(1.63426473152765,-0.373586846396559,-0.174042761838764));
#4332=CARTESIAN_POINT('Ctrl Pts',(1.62691869420078,-0.33909093068465,-0.233069203882014));
#4333=CARTESIAN_POINT('Ctrl Pts',(1.62252828437015,-0.317195968905306,-0.261368388670537));
#4334=CARTESIAN_POINT('Ctrl Pts',(1.61365775139403,-0.266264900654909,-0.311480544243686));
#4335=CARTESIAN_POINT('Ctrl Pts',(1.60919314384089,-0.237231147975234,-0.333298652394954));
#4336=CARTESIAN_POINT('Ctrl Pts',(1.60050712143809,-0.166543350814306,-0.373030350867485));
#4337=CARTESIAN_POINT('Ctrl Pts',(1.59665523941937,-0.123401821157026,-0.388626558458099));
#4338=CARTESIAN_POINT('Ctrl Pts',(1.59456899932179,-0.07938,-0.397005914195118));
#4339=CARTESIAN_POINT('Origin',(0.,-0.07938,0.));
#4340=CARTESIAN_POINT('Origin',(0.,-0.07938,0.));
#4341=CARTESIAN_POINT('Origin',(1.675,-0.07938,0.));
#4342=CARTESIAN_POINT('Origin',(1.675,0.,0.));
#4343=CARTESIAN_POINT('Origin',(1.675,-0.07938,0.));
#4344=CARTESIAN_POINT('Origin',(0.,-0.47628,0.));
#4345=CARTESIAN_POINT('Origin',(0.,-0.07938,0.));
#5505=UNCERTAINTY_MEASURE_WITH_UNIT(LENGTH_MEASURE(0.001),#5536,
'DISTANCE_ACCURACY_VALUE',
'Maximum model space distance between geometric entities at asserted c
onnectivities');
#5516=UNCERTAINTY_MEASURE_WITH_UNIT(LENGTH_MEASURE(0.001),#5536,
'DISTANCE_ACCURACY_VALUE',
'Maximum model space distance between geometric entities at asserted c
onnectivities');
#5524=(
GEOMETRIC_REPRESENTATION_CONTEXT(3)
GLOBAL_UNCERTAINTY_ASSIGNED_CONTEXT((#5505))
GLOBAL_UNIT_ASSIGNED_CONTEXT((#5536,#5538,#5539))
REPRESENTATION_CONTEXT('','3D')
);
#5535=(
GEOMETRIC_REPRESENTATION_CONTEXT(3)
GLOBAL_UNCERTAINTY_ASSIGNED_CONTEXT((#5516))
GLOBAL_UNIT_ASSIGNED_CONTEXT((#5536,#5538,#5539))
REPRESENTATION_CONTEXT('','3D')
);
#5536=(
LENGTH_UNIT()
NAMED_UNIT(*)
SI_UNIT(.CENTI.,.METRE.)
);
#5538=(
NAMED_UNIT(*)
PLANE_ANGLE_UNIT()
SI_UNIT($,.RADIAN.)
);
#5539=(
NAMED_UNIT(*)
SI_UNIT($,.STERADIAN.)
SOLID_ANGLE_UNIT()
);
#5547=SHAPE_DEFINITION_REPRESENTATION(#5565,#5608);
#5565=PRODUCT_DEFINITION_SHAPE('',$,#5627);
#5608=SHAPE_REPRESENTATION('',(#2623),#5524);
#5619=PRODUCT_DEFINITION_CONTEXT('part definition',#5675,'design');
#5627=PRODUCT_DEFINITION('Cage','Cage',#5645,#5619);
#5645=PRODUCT_DEFINITION_FORMATION('',$,#5684);
#5675=APPLICATION_CONTEXT(
'Core Data for Automotive Mechanical Design Process');
#5676=PRODUCT_CONTEXT('part definition',#5675,'mechanical');
#5684=PRODUCT('Cage','Cage','Cage',(#5676));
#5758=COLOUR_RGB('Grey',0.48,0.52,0.57);
#5759=FILL_AREA_STYLE_COLOUR('',#5758);
#5760=FILL_AREA_STYLE('',(#5759));
#5761=SURFACE_STYLE_FILL_AREA(#5760);
#5762=SURFACE_SIDE_STYLE('',(#5761));
#5763=SURFACE_STYLE_USAGE(.BOTH.,#5762);
#5764=PRESENTATION_STYLE_ASSIGNMENT((#5763));
ENDSEC;
END-ISO-10303-21;
